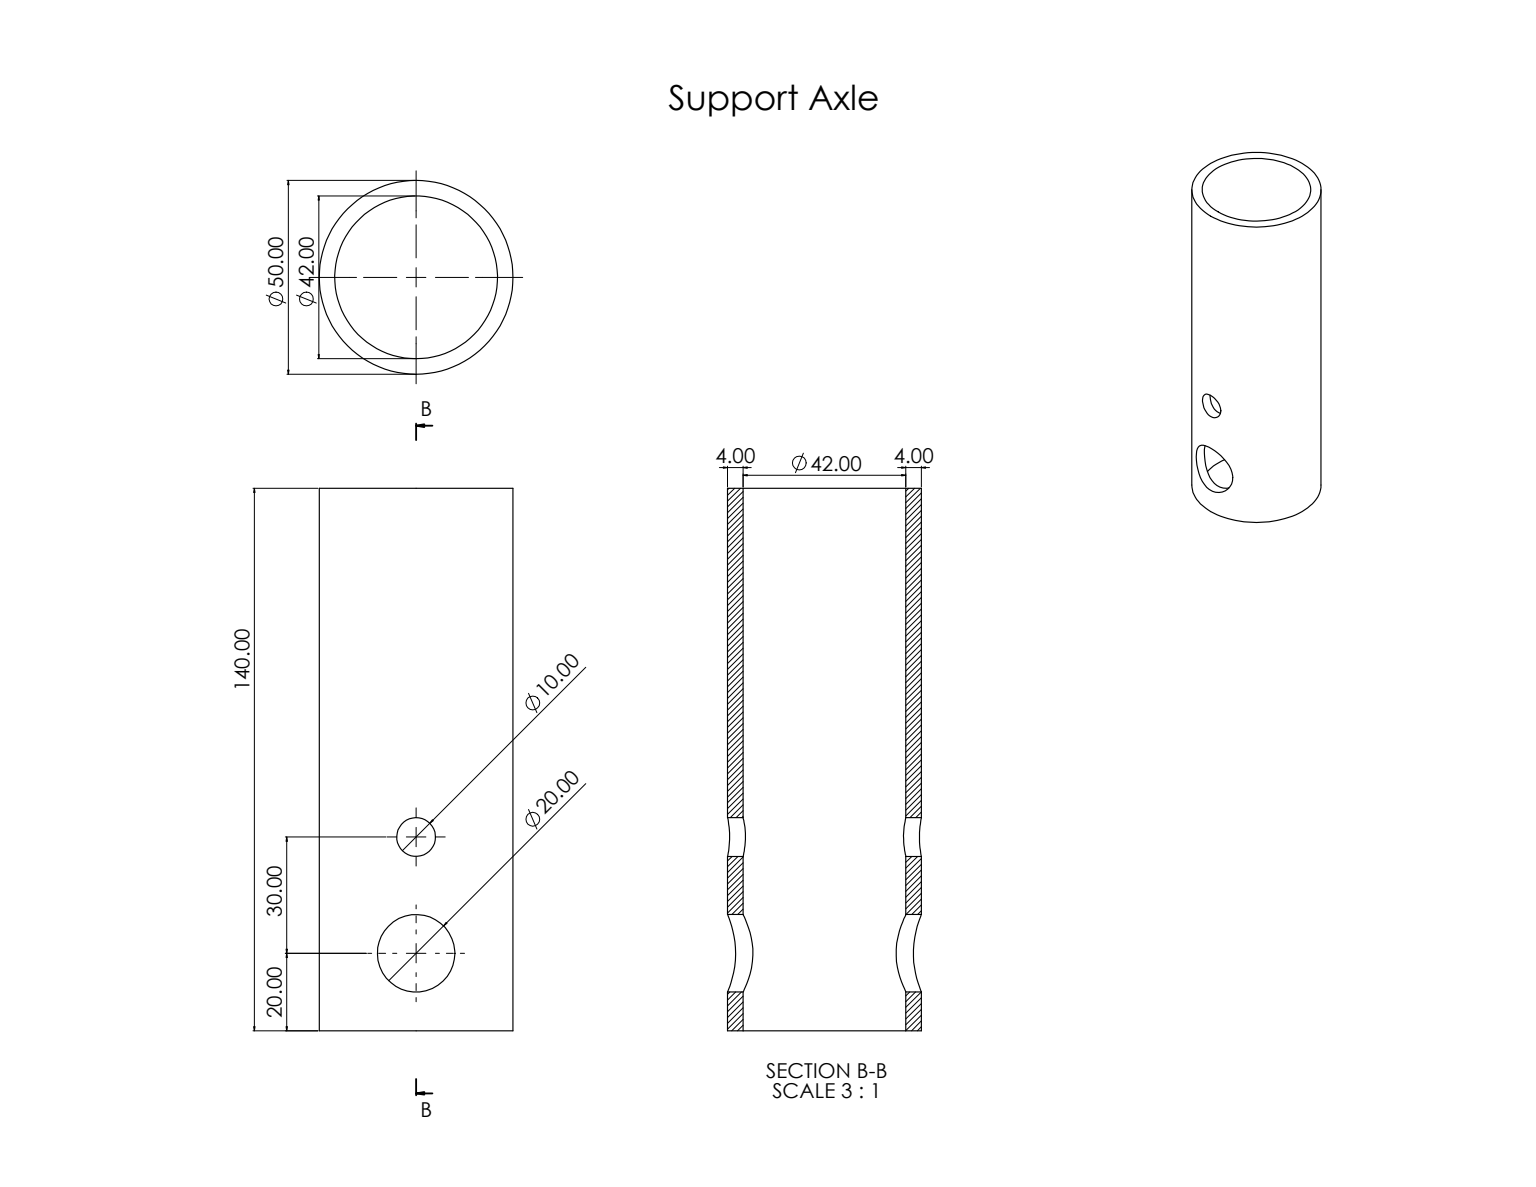
ISO-10303-21;
HEADER;
FILE_DESCRIPTION (('STEP AP214'),
    '1' );
FILE_NAME ('Support Axle.step',
    '2026-10-19T17:36:30',
    ( '' ),
    ( '' ),
    'SwSTEP 2.0',
    'SolidWorks 2025',
    '' );
FILE_SCHEMA (( 'AUTOMOTIVE_DESIGN' ));
ENDSEC;

DATA;
#26=CARTESIAN_POINT ( 'NONE',  ( 5.000000000000000888, 49.66980702654861801, -24.49489742783178059 ) ) ;
#42=CARTESIAN_POINT ( 'NONE',  ( -5.000000000000000000, 50.00000000000000000, 24.49489742783178414 ) ) ;
#55=CARTESIAN_POINT ( 'NONE',  ( 1.302272420532246455, 45.16122859629937381, -20.96210264449279137 ) ) ;
#72=DIRECTION ( 'NONE',  ( 0.000000000000000000, 0.000000000000000000, 1.000000000000000000 ) ) ;
#75=EDGE_CURVE ( 'NONE', #1856, #7546, #10580, .T. ) ;
#100=EDGE_CURVE ( 'NONE', #1932, #332, #3178, .T. ) ;
#104=CARTESIAN_POINT ( 'NONE',  ( -9.477880355945590196, 23.25612560302911902, 18.74165831626246970 ) ) ;
#120=CARTESIAN_POINT ( 'NONE',  ( -3.766911610146119305, 46.69571375074811925, -24.71569286637712892 ) ) ;
#139=EDGE_CURVE ( 'NONE', #6118, #11306, #5452, .T. ) ;
#141=EDGE_LOOP ( 'NONE', ( #2879, #8210, #6869, #7953, #8806, #9023 ) ) ;
#143=CARTESIAN_POINT ( 'NONE',  ( -3.767068525368503895, 53.30379312071067233, -24.71564595051174607 ) ) ;
#153=FACE_BOUND ( 'NONE', #206, .T. ) ;
#183=CARTESIAN_POINT ( 'NONE',  ( 4.999999999999999112, 49.83503777815744940, -20.39607805437113441 ) ) ;
#192=AXIS2_PLACEMENT_3D ( 'NONE', #3678, #11483, #9714 ) ;
#196=CIRCLE ( 'NONE', #3434, 25.00000000000000000 ) ;
#204=ORIENTED_EDGE ( 'NONE', *, *, #7341, .T. ) ;
#206=EDGE_LOOP ( 'NONE', ( #5971, #3892 ) ) ;
#207=DIRECTION ( 'NONE',  ( 1.000000000000000000, 0.000000000000000000, 0.000000000000000000 ) ) ;
#216=MECHANICAL_DESIGN_GEOMETRIC_PRESENTATION_REPRESENTATION('',(#1626),#7294);
#226=PRODUCT_DEFINITION_SHAPE ( 'NONE', 'NONE',  #5124 ) ;
#231=CARTESIAN_POINT ( 'NONE',  ( -10.00000000000000178, 20.33047844303349905, 18.46618531261938756 ) ) ;
#233=ORIENTED_EDGE ( 'NONE', *, *, #8654, .T. ) ;
#239=ORIENTED_EDGE ( 'NONE', *, *, #75, .F. ) ;
#252=CARTESIAN_POINT ( 'NONE',  ( 3.053062343563090142, 46.02672757820099037, 20.77871069257179215 ) ) ;
#281=CARTESIAN_POINT ( 'NONE',  ( 3.052678183968668524, 46.02654057254596154, -24.81443426854575307 ) ) ;
#289=PRODUCT_DEFINITION_CONTEXT ( 'detailed design', #1328, 'design' ) ;
#310=CARTESIAN_POINT ( 'NONE',  ( 8.648152576036682859, 25.03146049264868367, 19.13735728885347243 ) ) ;
#314=CARTESIAN_POINT ( 'NONE',  ( 3.974373595566621731, 46.94861671663893077, 20.62131536938402832 ) ) ;
#325=AXIS2_PLACEMENT_3D ( 'NONE', #1284, #11686, #5158 ) ;
#332=VERTEX_POINT ( 'NONE', #3766 ) ;
#349=ORIENTED_EDGE ( 'NONE', *, *, #10874, .F. ) ;
#355=CIRCLE ( 'NONE', #6829, 21.00000000000000000 ) ;
#360=ORIENTED_EDGE ( 'NONE', *, *, #5907, .F. ) ;
#369=CARTESIAN_POINT ( 'NONE',  ( 10.00000000000000533, 19.67046583110989744, -22.91287847477920181 ) ) ;
#373=DIRECTION ( 'NONE',  ( 0.000000000000000000, 0.000000000000000000, -1.000000000000000000 ) ) ;
#376=CARTESIAN_POINT ( 'NONE',  ( 3.260856397143627294, 29.47603743248158636, -20.75437471433135883 ) ) ;
#377=CARTESIAN_POINT ( 'NONE',  ( 1.612540704446980389, 45.26432593853714081, 20.93858753690425090 ) ) ;
#384=AXIS2_PLACEMENT_3D ( 'NONE', #11930, #5963, #3236 ) ;
#398=CARTESIAN_POINT ( 'NONE',  ( 2.571758278209441661E-15, 0.000000000000000000, 21.00000000000000000 ) ) ;
#426=ORIENTED_EDGE ( 'NONE', *, *, #9632, .F. ) ;
#427=CARTESIAN_POINT ( 'NONE',  ( -6.613021203892899713, 12.47133511838782383, -19.93742635182809053 ) ) ;
#428=CARTESIAN_POINT ( 'NONE',  ( -0.3295322344531997905, 30.00000000000001066, 25.00000000000001066 ) ) ;
#442=CARTESIAN_POINT ( 'NONE',  ( 3.974960981574284347, 46.94936902441865101, 24.68265737646872893 ) ) ;
#447=CARTESIAN_POINT ( 'NONE',  ( 0.000000000000000000, 139.9999999999999716, 0.000000000000000000 ) ) ;
#467=ORIENTED_EDGE ( 'NONE', *, *, #7068, .F. ) ;
#468=CYLINDRICAL_SURFACE ( 'NONE', #9354, 5.000000000000000000 ) ;
#489=CARTESIAN_POINT ( 'NONE',  ( 9.917674697986294419, 18.67684296126092747, -22.94866065126248600 ) ) ;
#494=CARTESIAN_POINT ( 'NONE',  ( 3.061616998149962604E-15, 10.00000000000000000, 25.00000000000000000 ) ) ;
#500=CARTESIAN_POINT ( 'NONE',  ( 2.612127725832936065, 29.65839247515747346, 24.86517017815632968 ) ) ;
#517=VECTOR ( 'NONE', #12407, 1000.000000000000000 ) ;
#529=CARTESIAN_POINT ( 'NONE',  ( -2.067585255946370548, 45.44456205236168245, 24.91481882275639848 ) ) ;
#544=ORIENTED_EDGE ( 'NONE', *, *, #6668, .F. ) ;
#548=CARTESIAN_POINT ( 'NONE',  ( -2.620496854523448604, 10.32661740714168097, -24.87086379260451707 ) ) ;
#550=CARTESIAN_POINT ( 'NONE',  ( 6.615773601782837687, 12.47291401044366310, -24.11353245396511014 ) ) ;
#555=DIRECTION ( 'NONE',  ( 1.000000000000000000, 0.000000000000000000, 0.000000000000000000 ) ) ;
#558=CARTESIAN_POINT ( 'NONE',  ( -1.614380680224908104, 54.74360302825979119, 24.94967786989446878 ) ) ;
#573=LINE ( 'NONE', #5584, #10338 ) ;
#597=LINE ( 'NONE', #3505, #11293 ) ;
#610=CARTESIAN_POINT ( 'NONE',  ( -7.514688383768903357, 13.39426057884744026, -23.84485093628785535 ) ) ;
#611=CARTESIAN_POINT ( 'NONE',  ( 2.620611987601386250, 10.32688167823381953, -24.87076294850758984 ) ) ;
#616=CARTESIAN_POINT ( 'NONE',  ( 5.000000000000000888, 50.00000000000000000, -20.39607805437114152 ) ) ;
#621=CARTESIAN_POINT ( 'NONE',  ( 4.444397983376138228, 28.96407317687630822, 24.60352964329958070 ) ) ;
#622=CARTESIAN_POINT ( 'NONE',  ( -4.839306774598123084, 51.30008082132634684, 24.52723862394605092 ) ) ;
#640=EDGE_CURVE ( 'NONE', #4818, #9118, #196, .T. ) ;
#646=CARTESIAN_POINT ( 'NONE',  ( -1.322110193236855746, 29.91777919888772885, 20.96095187701988394 ) ) ;
#653=CARTESIAN_POINT ( 'NONE',  ( 3.561025220032636440, 10.64985055133391079, 20.69813086000296209 ) ) ;
#666=( NAMED_UNIT ( * ) SI_UNIT ( $, .STERADIAN. ) SOLID_ANGLE_UNIT ( ) );
#670=CARTESIAN_POINT ( 'NONE',  ( -3.245616027290198602, 10.51897860477085622, -24.79588311023535852 ) ) ;
#671=CARTESIAN_POINT ( 'NONE',  ( 9.917815328463536417, 18.67816480429018711, -18.51049262088216807 ) ) ;
#677=CARTESIAN_POINT ( 'NONE',  ( 0.000000000000000000, 139.9999999999999716, 0.000000000000000000 ) ) ;
#705=CARTESIAN_POINT ( 'NONE',  ( -5.310537848405668448, 28.47956428665436235, 20.31934704339811049 ) ) ;
#723=CARTESIAN_POINT ( 'NONE',  ( -3.554546826686217020, 29.35267307038308360, -24.74790415999775917 ) ) ;
#731=CARTESIAN_POINT ( 'NONE',  ( 2.218782135151963431, 54.49261812855775844, 20.88465242318871873 ) ) ;
#741=CARTESIAN_POINT ( 'NONE',  ( 9.657343816332662811, 22.61594140643868300, 23.05962942824199757 ) ) ;
#746=CARTESIAN_POINT ( 'NONE',  ( -3.255620798467798060, 29.46102596484070446, -20.74857864660710405 ) ) ;
#747=EDGE_CURVE ( 'NONE', #3111, #7940, #4337, .T. ) ;
#769=CARTESIAN_POINT ( 'NONE',  ( -5.000000000000000000, 50.00000000000000000, -20.39607805437114152 ) ) ;
#772=CARTESIAN_POINT ( 'NONE',  ( 9.932934464065827029, 18.66923383145512005, 18.50293221336126237 ) ) ;
#775=CARTESIAN_POINT ( 'NONE',  ( -0.6569842770428546697, 54.96739046863824996, -24.99342020365237360 ) ) ;
#794=CARTESIAN_POINT ( 'NONE',  ( 6.113716319958878209, 12.07992478634019662, -20.09207169644096780 ) ) ;
#797=ADVANCED_FACE ( 'NONE', ( #11879 ), #3185, .F. ) ;
#808=CARTESIAN_POINT ( 'NONE',  ( 1.342157722727130131E-15, 30.00000000000002132, -21.00000000000000355 ) ) ;
#829=ORIENTED_EDGE ( 'NONE', *, *, #2173, .T. ) ;
#855=CARTESIAN_POINT ( 'NONE',  ( 0.6627065662273624591, 10.01637405127483049, -20.99218728179891613 ) ) ;
#859=CARTESIAN_POINT ( 'NONE',  ( -3.305497356469124792, 46.23421970496524125, 20.73954946919153031 ) ) ;
#866=CARTESIAN_POINT ( 'NONE',  ( 5.000000000000000888, 50.00000000000000000, -20.39607805437114152 ) ) ;
#872=CARTESIAN_POINT ( 'NONE',  ( 0.000000000000000000, 0.000000000000000000, 0.000000000000000000 ) ) ;
#877=CARTESIAN_POINT ( 'NONE',  ( -3.051621101708449579, 53.97419359098365987, -20.77889715443343377 ) ) ;
#878=CARTESIAN_POINT ( 'NONE',  ( 3.061616997868383043E-15, 139.9999999999999716, 25.00000000000000000 ) ) ;
#892=B_SPLINE_CURVE_WITH_KNOTS ( 'NONE', 3,
 ( #7213, #5385, #9191, #2454, #500, #2580, #12107, #6328, #621, #5570, #3473, #6450, #6268, #8421, #9439, #12291, #6510, #11087, #1687, #10141, #10312, #741, #4609, #5321, #1631, #4364, #9318, #8299 ),
 .UNSPECIFIED., .F., .F.,
 ( 4, 2, 2, 2, 2, 2, 2, 2, 2, 2, 2, 2, 2, 4 ),
 ( 0.04738593773884331589, 0.04935840384251231894, 0.05034463689434681699, 0.05133086994618132198, 0.05231710299801582004, 0.05330333604985031809, 0.05527580215351931420, 0.05626203520535381225, 0.05724826825718831030, 0.05922073436085731335, 0.06020696741269181834, 0.06119320046452632333, 0.06217943351636082833, 0.06316566656819533332 ),
 .UNSPECIFIED. ) ;
#917=CARTESIAN_POINT ( 'NONE',  ( 8.667518415056527203, 14.97026592263945410, 23.45254893740142066 ) ) ;
#924=CARTESIAN_POINT ( 'NONE',  ( 0.3308316500937774629, 9.999999999999994671, -21.00000000000000711 ) ) ;
#937=ORIENTED_EDGE ( 'NONE', *, *, #4287, .F. ) ;
#941=CARTESIAN_POINT ( 'NONE',  ( -4.473766101552917540, 28.96742557902637927, -20.52713491992151162 ) ) ;
#946=DIRECTION ( 'NONE',  ( -0.000000000000000000, -1.000000000000000000, -0.000000000000000000 ) ) ;
#950=CARTESIAN_POINT ( 'NONE',  ( 1.326742001580319741, 29.91711497655587948, -24.96694321103489855 ) ) ;
#951=UNCERTAINTY_MEASURE_WITH_UNIT (LENGTH_MEASURE( 1.000000000000000082E-05 ), #4583, 'distance_accuracy_value', 'NONE');
#958=EDGE_CURVE ( 'NONE', #8162, #11970, #11300, .T. ) ;
#963=ORIENTED_EDGE ( 'NONE', *, *, #640, .T. ) ;
#978=CARTESIAN_POINT ( 'NONE',  ( -6.849710128414980836, 27.29284600759404356, -24.04449974210336904 ) ) ;
#980=ORIENTED_EDGE ( 'NONE', *, *, #75, .T. ) ;
#982=CARTESIAN_POINT ( 'NONE',  ( 6.110979747148361341, 12.05740682582580625, 24.24803741642852373 ) ) ;
#985=EDGE_CURVE ( 'NONE', #8822, #6118, #9067, .T. ) ;
#987=FACE_OUTER_BOUND ( 'NONE', #9258, .T. ) ;
#1002=CARTESIAN_POINT ( 'NONE',  ( 3.975237584097107923, 53.05037957731131826, -20.62115343197593020 ) ) ;
#1016=CARTESIAN_POINT ( 'NONE',  ( 10.00000000000000178, 20.33006360438132987, -18.46618531261938756 ) ) ;
#1020=CARTESIAN_POINT ( 'NONE',  ( 6.844556472468130259, 27.29775667647069071, -24.04598060202682319 ) ) ;
#1044=DIRECTION ( 'NONE',  ( -0.000000000000000000, -1.000000000000000000, -0.000000000000000000 ) ) ;
#1059=CARTESIAN_POINT ( 'NONE',  ( -9.983660626454435416, 20.66196728388187864, 18.47506278258854806 ) ) ;
#1071=CARTESIAN_POINT ( 'NONE',  ( -5.000000000000000000, 50.00000000000000000, -24.49489742783178059 ) ) ;
#1072=CARTESIAN_POINT ( 'NONE',  ( 4.490871182873028111, 47.77729020916527958, -20.51460075614775036 ) ) ;
#1106=AXIS2_PLACEMENT_3D ( 'NONE', #12286, #5873, #10807 ) ;
#1109=CARTESIAN_POINT ( 'NONE',  ( 4.491542451266983704, 47.77873343313099497, -24.59354576118897739 ) ) ;
#1114=DIRECTION ( 'NONE',  ( 1.000000000000000000, 0.000000000000000000, 0.000000000000000000 ) ) ;
#1125=CARTESIAN_POINT ( 'NONE',  ( 4.999999999999999112, 50.32998418051842293, -24.49489742783177348 ) ) ;
#1130=ORIENTED_EDGE ( 'NONE', *, *, #3730, .T. ) ;
#1133=CYLINDRICAL_SURFACE ( 'NONE', #4793, 25.00000000000000000 ) ;
#1138=CARTESIAN_POINT ( 'NONE',  ( 9.477187959615639201, 23.25714206674319939, 18.74197276232252563 ) ) ;
#1144=CARTESIAN_POINT ( 'NONE',  ( 9.658351069856484727, 22.61227114741398836, -23.05920763558311037 ) ) ;
#1147=PRODUCT_CONTEXT ( 'NONE', #8453, 'mechanical' ) ;
#1174=EDGE_CURVE ( 'NONE', #8715, #3634, #892, .T. ) ;
#1176=CARTESIAN_POINT ( 'NONE',  ( 2.065847364689658683, 45.44381439048179772, -24.91495664786098274 ) ) ;
#1178=ORIENTED_EDGE ( 'NONE', *, *, #6560, .F. ) ;
#1199=DIRECTION ( 'NONE',  ( 0.000000000000000000, 0.000000000000000000, 1.000000000000000000 ) ) ;
#1202=CARTESIAN_POINT ( 'NONE',  ( 8.957304208062865314, 24.45789625178892734, 18.99462261546309705 ) ) ;
#1221=VERTEX_POINT ( 'NONE', #7338 ) ;
#1254=CARTESIAN_POINT ( 'NONE',  ( -4.158535434072708092, 10.89987024370912572, -20.58639742492232827 ) ) ;
#1259=CARTESIAN_POINT ( 'NONE',  ( 2.630514865864268970, 29.67066479083239372, 20.84486189436999837 ) ) ;
#1260=CARTESIAN_POINT ( 'NONE',  ( 3.975399702753076525, 46.95009918027220408, -20.62111044216656452 ) ) ;
#1265=ORIENTED_EDGE ( 'NONE', *, *, #2271, .T. ) ;
#1266=B_SPLINE_CURVE_WITH_KNOTS ( 'NONE', 3,
 ( #4749, #8741, #6707, #55, #8495, #2843, #5641, #3668, #10576, #1887, #1260, #9763, #1072, #5952, #10828, #9827, #6896, #11726, #183, #10761 ),
 .UNSPECIFIED., .F., .F.,
 ( 4, 2, 2, 2, 2, 2, 2, 2, 2, 4 ),
 ( 0.01568878760782931384, 0.01666929802245319808, 0.01764980843707708580, 0.01863031885170097005, 0.01961082926632485429, 0.02059133968094873854, 0.02157185009557262279, 0.02255236051019651050, 0.02304261571750846130, 0.02353287092482041556 ),
 .UNSPECIFIED. ) ;
#1280=ORIENTED_EDGE ( 'NONE', *, *, #3433, .T. ) ;
#1284=CARTESIAN_POINT ( 'NONE',  ( 0.000000000000000000, 20.00000000000000355, -28.00000000000000711 ) ) ;
#1297=CARTESIAN_POINT ( 'NONE',  ( 1.302738838705299829, 54.83847614797452508, -20.96203534374045674 ) ) ;
#1299=ORIENTED_EDGE ( 'NONE', *, *, #9071, .F. ) ;
#1319=CARTESIAN_POINT ( 'NONE',  ( -6.116903510341333394, 12.06222645458920084, -20.09722343790940613 ) ) ;
#1322=CARTESIAN_POINT ( 'NONE',  ( -8.658175568303594360, 14.98574592473889311, 23.45342671841680371 ) ) ;
#1324=CARTESIAN_POINT ( 'NONE',  ( -3.050580840359966128, 46.02510565206127779, -24.81467268664276560 ) ) ;
#1328=APPLICATION_CONTEXT ( 'automotive_design' ) ;
#1380=CARTESIAN_POINT ( 'NONE',  ( -7.294862588765995248, 13.15250477205630553, -19.69373592174549259 ) ) ;
#1412=ADVANCED_FACE ( 'NONE', ( #11714 ), #7907, .F. ) ;
#1441=DIRECTION ( 'NONE',  ( -0.000000000000000000, -1.000000000000000000, -0.000000000000000000 ) ) ;
#1444=CARTESIAN_POINT ( 'NONE',  ( -3.558434346354896416, 10.64888650799004033, -20.69856808805790038 ) ) ;
#1450=CARTESIAN_POINT ( 'NONE',  ( -9.463516830393745138, 16.75202061662974273, 18.74709386869566430 ) ) ;
#1455=VECTOR ( 'NONE', #6408, 1000.000000000000000 ) ;
#1480=DIRECTION ( 'NONE',  ( 0.000000000000000000, 0.000000000000000000, 1.000000000000000000 ) ) ;
#1482=VECTOR ( 'NONE', #5857, 1000.000000000000000 ) ;
#1498=CARTESIAN_POINT ( 'NONE',  ( -4.441326820874226478, 11.03441940688963108, -24.60408056175351987 ) ) ;
#1500=CARTESIAN_POINT ( 'NONE',  ( -9.103371648737914157, 24.15160165414906857, 23.28405058525132176 ) ) ;
#1506=CARTESIAN_POINT ( 'NONE',  ( -8.488010075893786421, 14.70289628708776242, 19.20917730135813528 ) ) ;
#1514=CARTESIAN_POINT ( 'NONE',  ( 3.298734236876446957, 53.76100060739371145, 24.78173945428942204 ) ) ;
#1536=AXIS2_PLACEMENT_3D ( 'NONE', #5941, #8037, #8854 ) ;
#1565=CARTESIAN_POINT ( 'NONE',  ( 8.486510062750307171, 14.70060591898896618, -23.51628241912814588 ) ) ;
#1593=AXIS2_PLACEMENT_3D ( 'NONE', #10131, #1441, #4352 ) ;
#1600=CARTESIAN_POINT ( 'NONE',  ( -1.614021781250221999, 45.25640150583762988, -20.94007668992154692 ) ) ;
#1604=( NAMED_UNIT ( * ) PLANE_ANGLE_UNIT ( ) SI_UNIT ( $, .RADIAN. ) );
#1621=CARTESIAN_POINT ( 'NONE',  ( 9.105349949761121664, 15.85277269881838258, -23.28327519851026040 ) ) ;
#1626=STYLED_ITEM('',(#12584),#2150);
#1628=CARTESIAN_POINT ( 'NONE',  ( -7.537341967019228761, 13.39683431484485965, 19.60665308794510864 ) ) ;
#1631=CARTESIAN_POINT ( 'NONE',  ( 9.916835782772588814, 21.32911185711201796, 22.94902338049798374 ) ) ;
#1676=ORIENTED_EDGE ( 'NONE', *, *, #10874, .T. ) ;
#1678=CARTESIAN_POINT ( 'NONE',  ( -8.664197377259947430, 14.96499702975700608, -23.45374477514955203 ) ) ;
#1679=CARTESIAN_POINT ( 'NONE',  ( 10.00000000000000711, 19.66959671226640793, -18.46618531261938756 ) ) ;
#1683=CARTESIAN_POINT ( 'NONE',  ( -0.3273843838414227103, 45.00000000000000711, 20.99999999999999645 ) ) ;
#1687=CARTESIAN_POINT ( 'NONE',  ( 8.972329510183547185, 24.46440230363330315, 23.33606587946024291 ) ) ;
#1722=CARTESIAN_POINT ( 'NONE',  ( -6.197539731915355238E-14, 9.999999999999182876, 21.00000000000039080 ) ) ;
#1740=CARTESIAN_POINT ( 'NONE',  ( 1.659095203930551543, 10.13304969779982301, -20.93688979605049738 ) ) ;
#1776=CARTESIAN_POINT ( 'NONE',  ( -5.000000000000000888, 49.67263425446288494, -20.39607805437114152 ) ) ;
#1778=B_SPLINE_CURVE_WITH_KNOTS ( 'NONE', 3,
 ( #9551, #9365, #8407, #9609, #6556, #8526, #9488, #5615, #917, #3576, #8650, #11322, #2629, #7578, #982, #4848, #9798, #6929, #4912, #1918, #8967, #8714, #6871, #3003 ),
 .UNSPECIFIED., .F., .F.,
 ( 4, 2, 2, 2, 2, 2, 2, 2, 2, 2, 2, 4 ),
 ( 0.000000000000000000, 0.001975470015275241145, 0.002963205022912861284, 0.003950940030550481423, 0.005926410045825732976, 0.006914145053463355284, 0.007901880061100976724, 0.009877350076376223073, 0.01185282009165146769, 0.01284055509928909086, 0.01382829010692671404, 0.01580376012220196039 ),
 .UNSPECIFIED. ) ;
#1779=CARTESIAN_POINT ( 'NONE',  ( 9.737577724063894991, 17.70041058371123555, 18.60604745661291659 ) ) ;
#1784=ADVANCED_FACE ( 'NONE', ( #6253 ), #5244, .T. ) ;
#1788=CARTESIAN_POINT ( 'NONE',  ( 5.000000000000000000, 50.00000000000000000, -24.49489742783178414 ) ) ;
#1827=FACE_OUTER_BOUND ( 'NONE', #6135, .T. ) ;
#1839=EDGE_LOOP ( 'NONE', ( #11508, #2743, #7233, #12183, #8498, #2835, #829, #9052, #10546, #10410, #9366, #12012, #9085, #9441, #6536, #8348 ) ) ;
#1843=CARTESIAN_POINT ( 'NONE',  ( 7.513991638149614793, 13.39363280574569792, 19.61093064431749156 ) ) ;
#1856=VERTEX_POINT ( 'NONE', #5970 ) ;
#1864=CARTESIAN_POINT ( 'NONE',  ( 3.061617454482527662E-15, 30.00000000000001066, 25.00000000000000000 ) ) ;
#1887=CARTESIAN_POINT ( 'NONE',  ( 3.765166081389465624, 46.69397311189987931, -20.66103212045354098 ) ) ;
#1918=CARTESIAN_POINT ( 'NONE',  ( 2.610381677634093123, 10.34108370468245219, 24.86537221636008965 ) ) ;
#1932=VERTEX_POINT ( 'NONE', #5056 ) ;
#1940=CARTESIAN_POINT ( 'NONE',  ( 4.492685090163540451, 52.21864068105092116, -20.51419621738226695 ) ) ;
#1948=CARTESIAN_POINT ( 'NONE',  ( -0.3317315395883421170, 55.00000000000000711, -21.00000000000000000 ) ) ;
#1967=AXIS2_PLACEMENT_3D ( 'NONE', #3895, #3202, #1114 ) ;
#1988=CARTESIAN_POINT ( 'NONE',  ( 0.000000000000000000, 139.9999999999999716, -25.00000000000000000 ) ) ;
#1993=CARTESIAN_POINT ( 'NONE',  ( -10.00000000000000355, 20.00000000000000355, 18.46618531261938756 ) ) ;
#2007=CARTESIAN_POINT ( 'NONE',  ( 0.000000000000000000, 0.000000000000000000, 0.000000000000000000 ) ) ;
#2011=CARTESIAN_POINT ( 'NONE',  ( 1.653699482248477182, 29.86790856825577478, 20.93734097219926582 ) ) ;
#2028=CIRCLE ( 'NONE', #12370, 25.00000000000000000 ) ;
#2044=VERTEX_POINT ( 'NONE', #5183 ) ;
#2061=ORIENTED_EDGE ( 'NONE', *, *, #4367, .F. ) ;
#2073=CARTESIAN_POINT ( 'NONE',  ( 2.636325768737970421, 29.66875067697592883, -20.84397515108148724 ) ) ;
#2078=CARTESIAN_POINT ( 'NONE',  ( 10.00000000000000355, 20.00000000000000355, -22.91287847477919826 ) ) ;
#2106=CARTESIAN_POINT ( 'NONE',  ( -10.00000000000000533, 20.66054119461773553, -22.91287847477919470 ) ) ;
#2109=AXIS2_PLACEMENT_3D ( 'NONE', #447, #4560, #11286 ) ;
#2124=EDGE_LOOP ( 'NONE', ( #4978, #8968, #10794, #2582, #3424, #204, #9766, #4611, #9474, #963, #4270, #1676, #233, #7725, #1265, #2770 ) ) ;
#2126=CARTESIAN_POINT ( 'NONE',  ( 2.221110608488543026, 54.49139573732541209, -24.90296241992962578 ) ) ;
#2140=CARTESIAN_POINT ( 'NONE',  ( 9.931121997304011018, 21.34393702597181530, 18.50391133509319630 ) ) ;
#2141=CARTESIAN_POINT ( 'NONE',  ( -1.614845647245295668, 54.74348708565381827, 20.94004496404980742 ) ) ;
#2145=CARTESIAN_POINT ( 'NONE',  ( 4.999999999999999112, 49.66826422043975242, 20.39607805437114507 ) ) ;
#2147=CARTESIAN_POINT ( 'NONE',  ( 9.104442389086463194, 24.14915179589751304, -23.28362858151144721 ) ) ;
#2150=MANIFOLD_SOLID_BREP ( 'Cut-Extrude1[1]', #9310 ) ;
#2166=CARTESIAN_POINT ( 'NONE',  ( -3.973726775714538029, 53.05247132632594287, -24.68286527305685141 ) ) ;
#2173=EDGE_CURVE ( 'NONE', #3634, #9164, #1778, .T. ) ;
#2180=EDGE_LOOP ( 'NONE', ( #6946, #7322, #9894, #5335, #11443, #10716 ) ) ;
#2181=CARTESIAN_POINT ( 'NONE',  ( 0.6582936873354101603, 54.96735637312282563, -20.99215814668205482 ) ) ;
#2186=LINE ( 'NONE', #1988, #5156 ) ;
#2201=EDGE_CURVE ( 'NONE', #2752, #10467, #5726, .T. ) ;
#2204=CARTESIAN_POINT ( 'NONE',  ( -9.461967865576259129, 16.74741879838144598, -18.74787822604630350 ) ) ;
#2211=CARTESIAN_POINT ( 'NONE',  ( 10.00000000000000355, 20.00000000000000355, 18.46618531261938401 ) ) ;
#2212=CARTESIAN_POINT ( 'NONE',  ( -2.222896043811084077, 54.49078271291326558, 20.88425106962813516 ) ) ;
#2217=CARTESIAN_POINT ( 'NONE',  ( 3.304159235005521111, 46.23328646880356274, 20.73974243245384841 ) ) ;
#2233=ORIENTED_EDGE ( 'NONE', *, *, #8936, .T. ) ;
#2234=ORIENTED_EDGE ( 'NONE', *, *, #3811, .T. ) ;
#2248=CARTESIAN_POINT ( 'NONE',  ( -3.304393266822325703, 46.23318141187127139, 24.78176792680001839 ) ) ;
#2268=CARTESIAN_POINT ( 'NONE',  ( -3.251483927478052482, 10.53766038749295753, -20.74918120701668300 ) ) ;
#2271=EDGE_CURVE ( 'NONE', #5152, #7013, #6332, .T. ) ;
#2274=CARTESIAN_POINT ( 'NONE',  ( -2.509809017951089682, 45.66333224303983229, -24.87518608377025231 ) ) ;
#2275=CARTESIAN_POINT ( 'NONE',  ( -0.3310653830415872800, 54.99172937625127133, 20.99802641299722339 ) ) ;
#2306=CARTESIAN_POINT ( 'NONE',  ( -5.000000000000000000, 50.00000000000000000, 24.49489742783178414 ) ) ;
#2318=B_SPLINE_CURVE_WITH_KNOTS ( 'NONE', 3,
 ( #11987, #4369, #3415, #7284, #2459, #6335, #10202, #9324, #8364, #1514, #8306, #12174, #3477, #7409, #6151, #2525, #5455, #10026, #8118, #6515 ),
 .UNSPECIFIED., .F., .F.,
 ( 4, 2, 2, 2, 2, 2, 2, 2, 2, 4 ),
 ( 0.02350813035260379893, 0.02448705762280033518, 0.02546598489299686796, 0.02644491216319340421, 0.02693437579829167233, 0.02742383943338994046, 0.02840276670358647670, 0.02938169397378300948, 0.03036062124397954226, 0.03133954851417607851 ),
 .UNSPECIFIED. ) ;
#2329=CARTESIAN_POINT ( 'NONE',  ( -7.519134213638725583, 26.60056234660722652, 23.84343405217310874 ) ) ;
#2333=DIRECTION ( 'NONE',  ( -0.000000000000000000, -0.000000000000000000, 1.000000000000000000 ) ) ;
#2335=CARTESIAN_POINT ( 'NONE',  ( -10.00000000000000355, 19.33860219128660063, 18.46618531261938045 ) ) ;
#2338=CARTESIAN_POINT ( 'NONE',  ( 2.506524500420500345, 45.66117316082983990, 20.85169879525578907 ) ) ;
#2364=VERTEX_POINT ( 'NONE', #3618 ) ;
#2385=CARTESIAN_POINT ( 'NONE',  ( -4.451684831872904091, 11.03962932791216112, -20.52483624935579343 ) ) ;
#2386=CARTESIAN_POINT ( 'NONE',  ( -5.303430480311382311, 28.48399989248413178, 24.43255084236253794 ) ) ;
#2388=CARTESIAN_POINT ( 'NONE',  ( -10.00000000000000355, 20.00000000000000355, 22.91287847477919826 ) ) ;
#2397=CARTESIAN_POINT ( 'NONE',  ( 0.3271393060908659445, 45.00000000000000711, 25.00000000000000355 ) ) ;
#2398=EDGE_CURVE ( 'NONE', #11698, #2695, #4652, .T. ) ;
#2424=CARTESIAN_POINT ( 'NONE',  ( -1.612909136089518691, 45.25592802960594696, 24.94976847917136453 ) ) ;
#2444=VERTEX_POINT ( 'NONE', #12444 ) ;
#2449=CARTESIAN_POINT ( 'NONE',  ( -9.869611566543289527, 18.35654797443324782, 22.96945393929722457 ) ) ;
#2454=CARTESIAN_POINT ( 'NONE',  ( 2.290457103807213457, 29.73981914200485477, 24.89699738223682246 ) ) ;
#2455=CARTESIAN_POINT ( 'NONE',  ( 0.000000000000000000, 139.9999999999999716, 0.000000000000000000 ) ) ;
#2458=CARTESIAN_POINT ( 'NONE',  ( 4.491750101222253377, 47.77928715861156661, 24.59350609687774281 ) ) ;
#2459=CARTESIAN_POINT ( 'NONE',  ( 1.614235646224727372, 54.74352724365349587, 24.94966740611544509 ) ) ;
#2466=B_SPLINE_CURVE_WITH_KNOTS ( 'NONE', 3,
 ( #11905, #1125, #8917, #7969, #3968, #6004, #8789, #8035, #6944, #7843, #5877, #3017, #10811, #6883, #2126, #7073, #6069, #9876, #5814, #4862 ),
 .UNSPECIFIED., .F., .F.,
 ( 4, 2, 2, 2, 2, 2, 2, 2, 2, 4 ),
 ( 0.02350824016915415912, 0.02448716854195917558, 0.02546609691476419204, 0.02644502528756920851, 0.02693448947397171500, 0.02742395366037422497, 0.02840288203317925531, 0.02938181040598428218, 0.03036073877878931251, 0.03133966715159434285 ),
 .UNSPECIFIED. ) ;
#2484=CARTESIAN_POINT ( 'NONE',  ( -3.051014581595654640, 46.02544827001062089, 24.81461801464184802 ) ) ;
#2493=B_SPLINE_CURVE_WITH_KNOTS ( 'NONE', 3,
 ( #8522, #3757, #6611, #4591, #9422, #9483, #723, #7637, #8463, #11502, #10544, #6046, #978, #7698, #6925, #10863, #4008, #8710, #8898, #7885, #10792, #5922, #2106, #12518 ),
 .UNSPECIFIED., .F., .F.,
 ( 4, 2, 2, 2, 2, 2, 2, 2, 2, 2, 2, 4 ),
 ( 5.438949063372056100E-19, 0.001975691086292785757, 0.002963536629439178418, 0.003951382172585572380, 0.005927073258878355969, 0.006914918802024747763, 0.007902764345171137822, 0.009878455431463928349, 0.01185414651775671888, 0.01284199206090311240, 0.01382983760404950767, 0.01580552869034228605 ),
 .UNSPECIFIED. ) ;
#2509=CARTESIAN_POINT ( 'NONE',  ( -10.00000000000000355, 20.00000000000000355, -22.91287847477919826 ) ) ;
#2511=CARTESIAN_POINT ( 'NONE',  ( -9.481431770954213079, 23.24517152888003224, 23.13387126485941536 ) ) ;
#2515=CARTESIAN_POINT ( 'NONE',  ( -1.652347697333065968, 10.13198208422932467, 24.94742907234073215 ) ) ;
#2524=VECTOR ( 'NONE', #4458, 1000.000000000000000 ) ;
#2525=CARTESIAN_POINT ( 'NONE',  ( 4.741482771685880948, 51.61996731904482516, 24.54657867284130646 ) ) ;
#2567=CARTESIAN_POINT ( 'NONE',  ( 0.6549955759030559044, 54.96769473000979644, 20.99223993983284586 ) ) ;
#2574=CARTESIAN_POINT ( 'NONE',  ( -5.000000000000000000, 49.67307781155022894, 20.39607805437114507 ) ) ;
#2575=CARTESIAN_POINT ( 'NONE',  ( -9.352703157270289225, 16.44582563935068009, 18.80282705866110149 ) ) ;
#2580=CARTESIAN_POINT ( 'NONE',  ( 3.239919941357241040, 29.46629152487073000, 24.79118428027058840 ) ) ;
#2581=CARTESIAN_POINT ( 'NONE',  ( -4.743460743378065558, 51.61424263853129446, 24.54619549801029166 ) ) ;
#2582=ORIENTED_EDGE ( 'NONE', *, *, #747, .T. ) ;
#2629=CARTESIAN_POINT ( 'NONE',  ( 7.297088297540795132, 13.15481214220262274, 23.91253034306283354 ) ) ;
#2635=CARTESIAN_POINT ( 'NONE',  ( 3.763812309688671753, 53.30741636328656341, 20.66126648110244801 ) ) ;
#2636=CARTESIAN_POINT ( 'NONE',  ( 9.670754941354928746, 17.37006389387946470, -18.64131299320824198 ) ) ;
#2640=DIRECTION ( 'NONE',  ( -0.000000000000000000, -1.000000000000000000, -0.000000000000000000 ) ) ;
#2647=ORIENTED_EDGE ( 'NONE', *, *, #10368, .T. ) ;
#2658=FACE_OUTER_BOUND ( 'NONE', #10327, .T. ) ;
#2675=CARTESIAN_POINT ( 'NONE',  ( 3.024050948510435495E-21, 45.00000000000000711, -21.00000000000000000 ) ) ;
#2677=CARTESIAN_POINT ( 'NONE',  ( 9.656537145003039058, 17.38065509551421073, 18.64841052569367719 ) ) ;
#2680=CARTESIAN_POINT ( 'NONE',  ( -0.3313438815916917579, 54.99999999999998579, -25.00000000000000000 ) ) ;
#2695=VERTEX_POINT ( 'NONE', #10589 ) ;
#2696=CARTESIAN_POINT ( 'NONE',  ( 4.967355519288257248, 50.65829285064151577, 20.40416061862378072 ) ) ;
#2697=CARTESIAN_POINT ( 'NONE',  ( 4.171089004654445986, 10.90545738055656066, -20.58391839369968324 ) ) ;
#2701=LINE ( 'NONE', #11336, #3226 ) ;
#2712=CARTESIAN_POINT ( 'NONE',  ( -10.00000000000000888, 20.66452866687815160, -18.46618531261939822 ) ) ;
#2720=CARTESIAN_POINT ( 'NONE',  ( -1.616912260125061618, 54.74267540711069557, -20.93986429502791324 ) ) ;
#2736=VERTEX_POINT ( 'NONE', #11163 ) ;
#2743=ORIENTED_EDGE ( 'NONE', *, *, #4161, .T. ) ;
#2744=DIRECTION ( 'NONE',  ( 0.000000000000000000, 0.000000000000000000, 1.000000000000000000 ) ) ;
#2752=VERTEX_POINT ( 'NONE', #8128 ) ;
#2769=CARTESIAN_POINT ( 'NONE',  ( 3.766346521502939471, 53.30452959794249068, -20.66080266315259806 ) ) ;
#2770=ORIENTED_EDGE ( 'NONE', *, *, #3384, .T. ) ;
#2773=CARTESIAN_POINT ( 'NONE',  ( -7.307805827056473191, 26.83368120074001695, -19.68893203084326515 ) ) ;
#2778=CARTESIAN_POINT ( 'NONE',  ( -1.298576428593012810, 54.83947011521958359, -20.96226629318544710 ) ) ;
#2799=CARTESIAN_POINT ( 'NONE',  ( 8.119414445536275338, 14.15357424190336566, 19.36786064314131650 ) ) ;
#2821=CARTESIAN_POINT ( 'NONE',  ( 8.484928971929276642, 14.69808267000900770, -19.21052728408403354 ) ) ;
#2826=CARTESIAN_POINT ( 'NONE',  ( -2.220931175283385350, 45.50830112210639555, 20.88445027029172962 ) ) ;
#2835=ORIENTED_EDGE ( 'NONE', *, *, #1174, .T. ) ;
#2839=PLANE ( 'NONE',  #8451 ) ;
#2843=CARTESIAN_POINT ( 'NONE',  ( 2.217630085887001279, 45.50684883240628409, -20.88476843860882326 ) ) ;
#2849=CARTESIAN_POINT ( 'NONE',  ( 8.654532730718658584, 25.02058024782134282, -23.45477484801500623 ) ) ;
#2879=ORIENTED_EDGE ( 'NONE', *, *, #11416, .F. ) ;
#2884=CARTESIAN_POINT ( 'NONE',  ( 9.478226885497544885, 16.74648819031018832, -18.74142151731972561 ) ) ;
#2906=CIRCLE ( 'NONE', #6153, 25.00000000000000000 ) ;
#2907=CARTESIAN_POINT ( 'NONE',  ( -3.307603021400832510, 53.76369073917810937, -20.73919124221722043 ) ) ;
#2937=CARTESIAN_POINT ( 'NONE',  ( 0.000000000000000000, 139.9999999999999716, 0.000000000000000000 ) ) ;
#2941=CARTESIAN_POINT ( 'NONE',  ( 4.337692624494786209, 47.49191884430658206, -24.62149689268095187 ) ) ;
#2972=CARTESIAN_POINT ( 'NONE',  ( -4.838792876751625727, 51.30218438880784504, 20.43503154247634868 ) ) ;
#2973=VECTOR ( 'NONE', #9723, 1000.000000000000000 ) ;
#2976=ORIENTED_EDGE ( 'NONE', *, *, #5725, .F. ) ;
#2977=EDGE_CURVE ( 'NONE', #1932, #1856, #573, .T. ) ;
#3003=CARTESIAN_POINT ( 'NONE',  ( 3.061616998149962604E-15, 10.00000000000000000, 25.00000000000000000 ) ) ;
#3017=CARTESIAN_POINT ( 'NONE',  ( 3.307338549894080604, 53.76391169785250668, -24.78134996739077422 ) ) ;
#3018=ORIENTED_EDGE ( 'NONE', *, *, #9369, .T. ) ;
#3030=CARTESIAN_POINT ( 'NONE',  ( 4.462445293788150025, 28.95508627606223229, 20.52252167446830100 ) ) ;
#3035=ORIENTED_EDGE ( 'NONE', *, *, #7930, .F. ) ;
#3036=CARTESIAN_POINT ( 'NONE',  ( -3.709758735690515970E-18, 30.00000000000001066, -25.00000000000000000 ) ) ;
#3067=CARTESIAN_POINT ( 'NONE',  ( 2.644456282953588921, 45.75339465611970269, -24.86012065554512063 ) ) ;
#3091=CARTESIAN_POINT ( 'NONE',  ( -0.8195736974120422236, 54.93507064933334050, 20.98461236856086032 ) ) ;
#3111=VERTEX_POINT ( 'NONE', #4133 ) ;
#3117=PRODUCT_DEFINITION_FORMATION_WITH_SPECIFIED_SOURCE ( 'ANY', '', #9041, .NOT_KNOWN. ) ;
#3129=CARTESIAN_POINT ( 'NONE',  ( 3.975724277407679974, 46.95046481276702366, -24.68253032026751370 ) ) ;
#3150=CARTESIAN_POINT ( 'NONE',  ( -8.118656623617184209, 14.15260872815194126, -19.36816941975095574 ) ) ;
#3152=CARTESIAN_POINT ( 'NONE',  ( 0.000000000000000000, 139.9999999999999716, 0.000000000000000000 ) ) ;
#3159=CARTESIAN_POINT ( 'NONE',  ( -1.612729787338046394, 45.25594143338945941, -24.94976830077123964 ) ) ;
#3160=CARTESIAN_POINT ( 'NONE',  ( -3.767196188295967918, 53.30371400289418915, 20.66066053404689029 ) ) ;
#3178=B_SPLINE_CURVE_WITH_KNOTS ( 'NONE', 3,
 ( #2509, #3464, #6561, #5501, #8288, #7520, #5560, #5374, #1678, #9370, #9245, #610, #12158, #11199, #7391, #10426, #11139, #1498, #3581, #670, #548, #4536, #6500, #4600, #7328, #3641 ),
 .UNSPECIFIED., .F., .F.,
 ( 4, 2, 2, 2, 2, 2, 2, 2, 2, 2, 2, 2, 4 ),
 ( 0.01580552869034228605, 0.01679261472842853362, 0.01777970076651477771, 0.01975387284268728671, 0.02172804491885978878, 0.02271513095694604328, 0.02370221699503229779, 0.02567638907120481373, 0.02666347510929107170, 0.02765056114737732967, 0.02962473322354984562, 0.03061181926163610706, 0.03159890529972236156 ),
 .UNSPECIFIED. ) ;
#3184=ORIENTED_EDGE ( 'NONE', *, *, #8798, .F. ) ;
#3185=CYLINDRICAL_SURFACE ( 'NONE', #325, 10.00000000000000355 ) ;
#3202=DIRECTION ( 'NONE',  ( -0.000000000000000000, -0.000000000000000000, 1.000000000000000000 ) ) ;
#3218=AXIS2_PLACEMENT_3D ( 'NONE', #5318, #9314, #373 ) ;
#3224=CARTESIAN_POINT ( 'NONE',  ( -4.968239015973206385, 50.65284130285913022, 20.40394647430411723 ) ) ;
#3226=VECTOR ( 'NONE', #2640, 1000.000000000000000 ) ;
#3228=CARTESIAN_POINT ( 'NONE',  ( 1.137587760790131908, 45.12834422743500085, 20.96978904175466596 ) ) ;
#3236=DIRECTION ( 'NONE',  ( 0.000000000000000000, 0.000000000000000000, 1.000000000000000000 ) ) ;
#3245=EDGE_CURVE ( 'NONE', #11306, #2044, #10375, .T. ) ;
#3255=CARTESIAN_POINT ( 'NONE',  ( -4.744071016079746350, 48.38731143956220393, 24.54607980264442091 ) ) ;
#3262=B_SPLINE_CURVE_WITH_KNOTS ( 'NONE', 3,
 ( #494, #4295, #6386, #4359, #2515, #11083, #4481, #3468, #8233, #3402, #6202, #11142, #7332, #5193, #3340, #5317, #1322, #9251, #7272, #6262, #4236, #2449, #6324, #8295, #10194, #2388 ),
 .UNSPECIFIED., .F., .F.,
 ( 4, 2, 2, 2, 2, 2, 2, 2, 2, 2, 2, 2, 4 ),
 ( 0.01580376012220196039, 0.01679085241551835084, 0.01777794470883474129, 0.01975212929546752219, 0.02172631388210030656, 0.02271340617541669701, 0.02370049846873308746, 0.02567468305536586837, 0.02666177534868225882, 0.02764886764199864927, 0.02962305222863143364, 0.03061014452194782409, 0.03159723681526421801 ),
 .UNSPECIFIED. ) ;
#3264=B_SPLINE_CURVE_WITH_KNOTS ( 'NONE', 3,
 ( #11410, #1948, #6583, #2778, #2720, #4685, #4619, #877, #2907, #4748, #8556, #6771, #8615, #10636, #11470, #4875, #3855, #12484, #3790, #10447 ),
 .UNSPECIFIED., .F., .F.,
 ( 4, 2, 2, 2, 2, 2, 2, 2, 2, 4 ),
 ( 3.491326639452381067E-19, 0.0009808062029949312765, 0.001961612405989862119, 0.002942418608984793179, 0.003923224811979723371, 0.004904031014974653997, 0.005884837217969585491, 0.006375240319467059477, 0.006865643420964533464, 0.007846449623959500519 ),
 .UNSPECIFIED. ) ;
#3278=ORIENTED_EDGE ( 'NONE', *, *, #4367, .T. ) ;
#3280=CARTESIAN_POINT ( 'NONE',  ( -8.651571107376318182, 25.02565239439968536, 23.45586713013333124 ) ) ;
#3286=CARTESIAN_POINT ( 'NONE',  ( 2.562745747226488176E-15, 30.00000000000001066, 21.00000000000000000 ) ) ;
#3289=CARTESIAN_POINT ( 'NONE',  ( 0.6529056306158902423, 45.03187583116404369, 20.99234021528525318 ) ) ;
#3313=VECTOR ( 'NONE', #946, 1000.000000000000000 ) ;
#3330=ORIENTED_EDGE ( 'NONE', *, *, #3811, .F. ) ;
#3337=CARTESIAN_POINT ( 'NONE',  ( -8.659888037695356644, 14.95771684574014948, -19.13532407230401944 ) ) ;
#3338=CARTESIAN_POINT ( 'NONE',  ( -2.619138840591237472, 29.67330545628644600, 24.87083797681799169 ) ) ;
#3340=CARTESIAN_POINT ( 'NONE',  ( -7.945999201647152788, 13.89399703635140249, 23.70671076423498391 ) ) ;
#3343=CARTESIAN_POINT ( 'NONE',  ( -6.197539731915355238E-14, 9.999999999999182876, 21.00000000000039080 ) ) ;
#3368=CARTESIAN_POINT ( 'NONE',  ( -6.197539731915355238E-14, 9.999999999999182876, 21.00000000000039080 ) ) ;
#3384=EDGE_CURVE ( 'NONE', #7013, #9272, #4628, .T. ) ;
#3398=CARTESIAN_POINT ( 'NONE',  ( 5.000000000000000000, 50.00000000000000000, 20.39607805437114152 ) ) ;
#3399=CARTESIAN_POINT ( 'NONE',  ( -6.109221465413982699, 27.94329460785578689, 24.24832107967536388 ) ) ;
#3401=EDGE_CURVE ( 'NONE', #11790, #4895, #2028, .T. ) ;
#3402=CARTESIAN_POINT ( 'NONE',  ( -5.845694806184612347, 11.88009017893230990, 24.30851799965319060 ) ) ;
#3404=CARTESIAN_POINT ( 'NONE',  ( -4.478749722781300235, 11.03480093803115558, 20.52614747825679942 ) ) ;
#3410=VERTEX_POINT ( 'NONE', #6511 ) ;
#3415=CARTESIAN_POINT ( 'NONE',  ( 0.6550203249928933102, 54.96765362015771927, 24.99347278016167095 ) ) ;
#3424=ORIENTED_EDGE ( 'NONE', *, *, #12017, .T. ) ;
#3433=EDGE_CURVE ( 'NONE', #10935, #2736, #5699, .T. ) ;
#3434=AXIS2_PLACEMENT_3D ( 'NONE', #5669, #12449, #9538 ) ;
#3440=CARTESIAN_POINT ( 'NONE',  ( -7.515231585295850891, 26.60501645963920225, 19.61046409729162932 ) ) ;
#3464=CARTESIAN_POINT ( 'NONE',  ( -10.00000000000000355, 19.66998333124466214, -22.91287847477919826 ) ) ;
#3465=CARTESIAN_POINT ( 'NONE',  ( -1.002883791299520887E-19, 10.00000000000000000, -25.00000000000000000 ) ) ;
#3468=CARTESIAN_POINT ( 'NONE',  ( -4.466051270639568749, 11.02833005318139925, 24.60558887372674519 ) ) ;
#3471=CYLINDRICAL_SURFACE ( 'NONE', #12424, 5.000000000000000000 ) ;
#3473=CARTESIAN_POINT ( 'NONE',  ( 5.303296350723960551, 28.48414319546200346, 24.43259468344301055 ) ) ;
#3476=CARTESIAN_POINT ( 'NONE',  ( 2.505975641493357831, 45.66085398937747186, 24.87560495202607669 ) ) ;
#3477=CARTESIAN_POINT ( 'NONE',  ( 3.971273688083300613, 53.05572982463418441, 24.68326415769028159 ) ) ;
#3494=CARTESIAN_POINT ( 'NONE',  ( -6.612279285637575832, 27.52949341102648262, 19.93770914801777749 ) ) ;
#3505=CARTESIAN_POINT ( 'NONE',  ( 10.00000000000000355, 20.00000000000000355, -28.00000000000000711 ) ) ;
#3512=CARTESIAN_POINT ( 'NONE',  ( 0.000000000000000000, 139.9999999999999716, -25.00000000000000000 ) ) ;
#3520=CARTESIAN_POINT ( 'NONE',  ( 1.648701702613829090, 10.13131270077370338, -24.94769321807935825 ) ) ;
#3526=CARTESIAN_POINT ( 'NONE',  ( -5.049704742916529376, 11.34434628041953452, 20.39145111578409697 ) ) ;
#3536=( GEOMETRIC_REPRESENTATION_CONTEXT ( 3 ) GLOBAL_UNCERTAINTY_ASSIGNED_CONTEXT ( ( #951 ) ) GLOBAL_UNIT_ASSIGNED_CONTEXT ( ( #4583, #1604, #3625 ) ) REPRESENTATION_CONTEXT ( 'NONE', 'WORKASPACE' ) );
#3543=CARTESIAN_POINT ( 'NONE',  ( -5.000000000000000000, 50.00000000000000000, -20.39607805437114152 ) ) ;
#3548=DIRECTION ( 'NONE',  ( -0.000000000000000000, -1.000000000000000000, -0.000000000000000000 ) ) ;
#3562=CARTESIAN_POINT ( 'NONE',  ( 2.295021694196371698, 10.26129700091049557, 20.87675788803829846 ) ) ;
#3572=DIRECTION ( 'NONE',  ( -0.000000000000000000, -0.000000000000000000, 1.000000000000000000 ) ) ;
#3576=CARTESIAN_POINT ( 'NONE',  ( 8.123360751522579193, 14.15902104166613107, 23.64419573351483450 ) ) ;
#3581=CARTESIAN_POINT ( 'NONE',  ( -4.146974088394097535, 10.89458658634673327, -24.65552811365946440 ) ) ;
#3589=DIRECTION ( 'NONE',  ( 0.000000000000000000, 1.000000000000000000, 0.000000000000000000 ) ) ;
#3593=CARTESIAN_POINT ( 'NONE',  ( -4.331872009808981794, 52.50234731214368367, 24.62196273622729592 ) ) ;
#3604=AXIS2_PLACEMENT_3D ( 'NONE', #9394, #10516, #7356 ) ;
#3618=CARTESIAN_POINT ( 'NONE',  ( -5.000000000000000000, 50.00000000000000000, 20.39607805437114152 ) ) ;
#3625=( NAMED_UNIT ( * ) SI_UNIT ( $, .STERADIAN. ) SOLID_ANGLE_UNIT ( ) );
#3627=ADVANCED_FACE ( 'NONE', ( #11184 ), #468, .F. ) ;
#3634=VERTEX_POINT ( 'NONE', #10114 ) ;
#3641=CARTESIAN_POINT ( 'NONE',  ( -1.002883791299520887E-19, 10.00000000000000000, -25.00000000000000000 ) ) ;
#3642=EDGE_CURVE ( 'NONE', #8125, #8822, #3658, .T. ) ;
#3658=CIRCLE ( 'NONE', #6307, 21.00000000000000000 ) ;
#3659=CARTESIAN_POINT ( 'NONE',  ( -9.657265040632822206, 22.61657440465215174, -18.64803156764659775 ) ) ;
#3660=DIRECTION ( 'NONE',  ( 0.000000000000000000, -0.000000000000000000, 1.000000000000000000 ) ) ;
#3668=CARTESIAN_POINT ( 'NONE',  ( 3.053082855025198494, 46.02690843307048141, -20.77868449535670692 ) ) ;
#3678=CARTESIAN_POINT ( 'NONE',  ( 0.000000000000000000, 50.00000000000000000, -28.00000000000000711 ) ) ;
#3686=CARTESIAN_POINT ( 'NONE',  ( -1.297374591076399408, 54.83977433137422253, -24.96837001061641104 ) ) ;
#3705=CARTESIAN_POINT ( 'NONE',  ( -4.493239192008157801, 47.78244187540930454, 20.51407495533472414 ) ) ;
#3730=EDGE_CURVE ( 'NONE', #5701, #7957, #9795, .T. ) ;
#3732=B_SPLINE_CURVE_WITH_KNOTS ( 'NONE', 3,
 ( #1993, #231, #1059, #8913, #5874, #4922, #104, #6940, #3964, #7965, #11833, #5409, #12132, #3440, #12254, #3494, #10223, #705, #11177, #5477, #6476, #9344, #10402, #9403, #646, #8980, #8031, #8446 ),
 .UNSPECIFIED., .F., .F.,
 ( 4, 2, 2, 2, 2, 2, 2, 2, 2, 2, 2, 2, 2, 4 ),
 ( 0.03175036704783668062, 0.03274152275842889814, 0.03373267846902110872, 0.03571498989020553683, 0.03670614560079775435, 0.03769730131138997187, 0.03868845702198218245, 0.03967961273257439997, 0.04166192415375883501, 0.04265307986435105253, 0.04364423557494327005, 0.04562654699612770509, 0.04661770270671992261, 0.04760885841731214013 ),
 .UNSPECIFIED. ) ;
#3757=CARTESIAN_POINT ( 'NONE',  ( -0.6685289520415670372, 30.00000000000001776, -25.00000000000001066 ) ) ;
#3766=CARTESIAN_POINT ( 'NONE',  ( -1.002883791299520887E-19, 10.00000000000000000, -25.00000000000000000 ) ) ;
#3771=CARTESIAN_POINT ( 'NONE',  ( -4.838567600861090057, 48.69772713945680209, 20.43508361496535031 ) ) ;
#3776=ORIENTED_EDGE ( 'NONE', *, *, #8676, .F. ) ;
#3782=CARTESIAN_POINT ( 'NONE',  ( -7.523626141222965025, 26.59539293290133344, -19.60723250985141775 ) ) ;
#3790=CARTESIAN_POINT ( 'NONE',  ( -4.999999999999999112, 50.32753737931852100, -20.39607805437113797 ) ) ;
#3795=CARTESIAN_POINT ( 'NONE',  ( 2.294321452706637121, 29.73876067080973229, -24.89658462890612967 ) ) ;
#3809=CARTESIAN_POINT ( 'NONE',  ( 6.843587254644259765, 12.70147400874256505, 19.85506230137591999 ) ) ;
#3811=EDGE_CURVE ( 'NONE', #3410, #7937, #11162, .T. ) ;
#3828=ORIENTED_EDGE ( 'NONE', *, *, #6489, .F. ) ;
#3855=CARTESIAN_POINT ( 'NONE',  ( -4.871666279273695999, 51.13754189277828743, -20.42713785987348984 ) ) ;
#3857=CARTESIAN_POINT ( 'NONE',  ( 9.918037823481203219, 21.32003297329905678, -18.51037319129331848 ) ) ;
#3880=LINE ( 'NONE', #10662, #1482 ) ;
#3885=DIRECTION ( 'NONE',  ( 0.000000000000000000, 1.000000000000000000, 0.000000000000000000 ) ) ;
#3892=ORIENTED_EDGE ( 'NONE', *, *, #5126, .F. ) ;
#3895=CARTESIAN_POINT ( 'NONE',  ( 0.000000000000000000, 20.00000000000000355, -28.00000000000000711 ) ) ;
#3918=CARTESIAN_POINT ( 'NONE',  ( -0.6578846949584694626, 54.95924935667866862, 20.99032885061396314 ) ) ;
#3950=FACE_OUTER_BOUND ( 'NONE', #9660, .T. ) ;
#3959=CYLINDRICAL_SURFACE ( 'NONE', #1967, 10.00000000000000355 ) ;
#3964=CARTESIAN_POINT ( 'NONE',  ( -8.955040573717580443, 24.46236383193878083, 18.99568595680172578 ) ) ;
#3968=CARTESIAN_POINT ( 'NONE',  ( 4.743537283058001819, 51.61420199850529400, -24.54618281552716041 ) ) ;
#3972=ORIENTED_EDGE ( 'NONE', *, *, #958, .T. ) ;
#4001=CARTESIAN_POINT ( 'NONE',  ( -3.050747483057216769, 53.97487283205587261, -24.81466456749452831 ) ) ;
#4008=CARTESIAN_POINT ( 'NONE',  ( -8.980220477185385519, 24.44733350940715866, -23.33298399582670157 ) ) ;
#4011=VERTEX_POINT ( 'NONE', #9273 ) ;
#4028=ORIENTED_EDGE ( 'NONE', *, *, #2398, .F. ) ;
#4041=CARTESIAN_POINT ( 'NONE',  ( -0.3266958997752330562, 45.00000000000001421, -25.00000000000000355 ) ) ;
#4042=CARTESIAN_POINT ( 'NONE',  ( -3.973286137925955863, 53.05282384735495782, 20.62152687101385951 ) ) ;
#4048=CARTESIAN_POINT ( 'NONE',  ( 5.034037828167091000, 28.66467738801596354, -24.49412005228846922 ) ) ;
#4098=CARTESIAN_POINT ( 'NONE',  ( -10.00000000000000355, 20.00000000000000355, -18.46618531261938401 ) ) ;
#4104=CARTESIAN_POINT ( 'NONE',  ( -4.484481976314367735, 47.78274414339135490, -24.59462526944309246 ) ) ;
#4132=CARTESIAN_POINT ( 'NONE',  ( -4.999999999999999112, 50.32713193883511593, -24.49489742783179125 ) ) ;
#4133=CARTESIAN_POINT ( 'NONE',  ( 5.340684424226280325E-17, 55.00000000000000000, -25.00000000000000000 ) ) ;
#4147=CARTESIAN_POINT ( 'NONE',  ( 2.222400765636041164, 54.49077458862202405, -20.88425590885463379 ) ) ;
#4161=EDGE_CURVE ( 'NONE', #11790, #9272, #9520, .T. ) ;
#4166=CARTESIAN_POINT ( 'NONE',  ( -9.983226034450831676, 19.33178880168245328, -18.47529793303663936 ) ) ;
#4175=EDGE_CURVE ( 'NONE', #5701, #3634, #6587, .T. ) ;
#4176=CARTESIAN_POINT ( 'NONE',  ( 1.342157722727130131E-15, 30.00000000000002132, -21.00000000000000355 ) ) ;
#4198=B_SPLINE_CURVE_WITH_KNOTS ( 'NONE', 3,
 ( #2078, #4819, #5008, #11671, #1144, #9705, #5898, #2147, #4941, #2849, #9896, #11733, #9643, #1020, #8745, #6776, #10642, #4048, #8807, #10834, #5773, #7926, #3795, #4881, #950, #11602, #8685, #3036 ),
 .UNSPECIFIED., .F., .F.,
 ( 4, 2, 2, 2, 2, 2, 2, 2, 2, 2, 2, 2, 2, 4 ),
 ( 0.04738924854463780201, 0.04936272659091893444, 0.05034946561405949372, 0.05133620463720005994, 0.05232294366034062616, 0.05330968268348119238, 0.05528316072976231788, 0.05626989975290288409, 0.05725663877604345031, 0.05923011682232458969, 0.06021685584546515591, 0.06120359486860571518, 0.06219033389174628140, 0.06317707291488684762 ),
 .UNSPECIFIED. ) ;
#4206=VECTOR ( 'NONE', #7834, 1000.000000000000000 ) ;
#4217=ADVANCED_FACE ( 'NONE', ( #1827 ), #6646, .F. ) ;
#4232=CARTESIAN_POINT ( 'NONE',  ( 10.00000000000000355, 20.00000000000000355, -22.91287847477919826 ) ) ;
#4236=CARTESIAN_POINT ( 'NONE',  ( -9.673562854105167474, 17.38029584746389133, 23.05303382818504332 ) ) ;
#4238=CARTESIAN_POINT ( 'NONE',  ( 6.119794236291119738, 27.93508701313207609, 20.09620109607250527 ) ) ;
#4251=CARTESIAN_POINT ( 'NONE',  ( 2.559760333650129958E-15, 55.00000000000000000, 21.00000000000000000 ) ) ;
#4270=ORIENTED_EDGE ( 'NONE', *, *, #6526, .F. ) ;
#4287=EDGE_CURVE ( 'NONE', #12540, #6613, #4198, .T. ) ;
#4290=CARTESIAN_POINT ( 'NONE',  ( -4.448741964560915640, 28.96190946584970405, 24.60274125495980613 ) ) ;
#4295=CARTESIAN_POINT ( 'NONE',  ( -0.3301927727158289749, 10.00000000000000000, 25.00000000000000355 ) ) ;
#4297=CARTESIAN_POINT ( 'NONE',  ( -7.945225341866328783, 13.89296426715405453, 19.44295823276161173 ) ) ;
#4299=CARTESIAN_POINT ( 'NONE',  ( 7.520704636030203893, 26.59870071877557507, -19.60835093631877513 ) ) ;
#4303=CARTESIAN_POINT ( 'NONE',  ( 3.052604782738682854, 46.02637368922790984, 24.81445626415020200 ) ) ;
#4337=B_SPLINE_CURVE_WITH_KNOTS ( 'NONE', 3,
 ( #8578, #2680, #775, #3686, #8891, #8007, #11808, #4001, #9849, #143, #2166, #8823, #6105, #8072, #10722, #7046, #4132, #6038 ),
 .UNSPECIFIED., .F., .F.,
 ( 4, 2, 2, 2, 2, 2, 2, 2, 4 ),
 ( 5.188175463412582976E-20, 0.0009797360301013575360, 0.001959472060202715072, 0.002939208090304072825, 0.003918944120405430144, 0.004898680150506787463, 0.005878416180608145650, 0.006858152210709502969, 0.007837888240810860288 ),
 .UNSPECIFIED. ) ;
#4344=VECTOR ( 'NONE', #3572, 1000.000000000000000 ) ;
#4352=DIRECTION ( 'NONE',  ( 0.000000000000000000, 0.000000000000000000, -1.000000000000000000 ) ) ;
#4355=CARTESIAN_POINT ( 'NONE',  ( 3.304769568038884664, 53.76613650905855479, 20.73964112051737274 ) ) ;
#4359=CARTESIAN_POINT ( 'NONE',  ( -1.325835098444672733, 10.08270123135439711, 24.96701611100131402 ) ) ;
#4364=CARTESIAN_POINT ( 'NONE',  ( 9.983143436873248788, 20.66859359106200955, 22.92025639428880623 ) ) ;
#4367=EDGE_CURVE ( 'NONE', #2044, #4011, #12050, .T. ) ;
#4369=CARTESIAN_POINT ( 'NONE',  ( 0.3299754220453550713, 55.00000000000001421, 25.00000000000000000 ) ) ;
#4389=CARTESIAN_POINT ( 'NONE',  ( -2.217326200926027724, 45.51555228448187762, 24.90189708455264395 ) ) ;
#4412=CARTESIAN_POINT ( 'NONE',  ( 7.537524037383855458, 13.39612119810769819, -23.84148986838564710 ) ) ;
#4418=CARTESIAN_POINT ( 'NONE',  ( -9.102716943808436767, 15.84719902056293250, 18.92511310367350319 ) ) ;
#4421=CARTESIAN_POINT ( 'NONE',  ( -2.221358530307614654, 54.49149874209361144, 24.90297606857491175 ) ) ;
#4454=CARTESIAN_POINT ( 'NONE',  ( -4.999999999999999112, 49.67330453822126657, 24.49489742783177348 ) ) ;
#4458=DIRECTION ( 'NONE',  ( -0.000000000000000000, -1.000000000000000000, -0.000000000000000000 ) ) ;
#4477=CARTESIAN_POINT ( 'NONE',  ( 3.246557057937244029, 10.51899376542992925, -24.79585947768713439 ) ) ;
#4481=CARTESIAN_POINT ( 'NONE',  ( -3.246935905771412667, 10.51876153604172970, 24.79592758899451255 ) ) ;
#4486=CARTESIAN_POINT ( 'NONE',  ( -4.246666789336575931, 52.64435674096336015, 24.63684932116156645 ) ) ;
#4488=CARTESIAN_POINT ( 'NONE',  ( 3.764226701178052803, 46.69296989397847852, 24.71608072572789538 ) ) ;
#4533=ORIENTED_EDGE ( 'NONE', *, *, #3245, .F. ) ;
#4536=CARTESIAN_POINT ( 'NONE',  ( -1.643512924178977430, 10.13039013404520716, -24.94805769307042453 ) ) ;
#4551=CARTESIAN_POINT ( 'NONE',  ( 1.298299055536097368, 45.16027954822755675, 24.96835849755778014 ) ) ;
#4560=DIRECTION ( 'NONE',  ( -0.000000000000000000, -1.000000000000000000, -0.000000000000000000 ) ) ;
#4583=( LENGTH_UNIT ( ) NAMED_UNIT ( * ) SI_UNIT ( .MILLI., .METRE. ) );
#4591=CARTESIAN_POINT ( 'NONE',  ( -2.290944097510326571, 29.73958545346254922, -24.89690719708686828 ) ) ;
#4600=CARTESIAN_POINT ( 'NONE',  ( -0.6576044892141179599, 10.01619439626406383, -24.99350884773162207 ) ) ;
#4605=CARTESIAN_POINT ( 'NONE',  ( -1.614219986190975620, 45.25635288715552207, 20.94008338602824182 ) ) ;
#4609=CARTESIAN_POINT ( 'NONE',  ( 9.737811142203947057, 22.29842083447240597, 23.02563804066124931 ) ) ;
#4611=ORIENTED_EDGE ( 'NONE', *, *, #100, .T. ) ;
#4619=CARTESIAN_POINT ( 'NONE',  ( -2.508870892452910173, 54.33730018467829126, -20.85139144392807253 ) ) ;
#4628=B_SPLINE_CURVE_WITH_KNOTS ( 'NONE', 3,
 ( #5512, #10438, #8483, #622, #2581, #9320, #7278, #3593, #4486, #11149, #5630, #12108, #9379, #10256, #4421, #558, #8361, #5447, #12354, #12292 ),
 .UNSPECIFIED., .F., .F.,
 ( 4, 2, 2, 2, 2, 2, 2, 2, 2, 4 ),
 ( 0.01567180661725443153, 0.01665134708417310289, 0.01763088755109177425, 0.01812065778455110993, 0.01861042801801044561, 0.01958996848492911697, 0.02056950895184778833, 0.02154904941876645622, 0.02252858988568512758, 0.02350813035260379893 ),
 .UNSPECIFIED. ) ;
#4629=VECTOR ( 'NONE', #2333, 1000.000000000000000 ) ;
#4638=CARTESIAN_POINT ( 'NONE',  ( -3.302322679538425287, 46.23143709543641933, -20.74005723812733848 ) ) ;
#4641=CARTESIAN_POINT ( 'NONE',  ( 7.297852186526522900, 13.15569421923598448, 19.69262651265845676 ) ) ;
#4646=CARTESIAN_POINT ( 'NONE',  ( 3.061616997868383043E-15, 0.000000000000000000, 25.00000000000000000 ) ) ;
#4652=B_SPLINE_CURVE_WITH_KNOTS ( 'NONE', 3,
 ( #769, #1776, #7624, #5660, #5723, #7498, #8509, #8573, #7370, #4638, #9408, #12259, #12384, #1600, #10465, #10406, #11487, #2675 ),
 .UNSPECIFIED., .F., .F.,
 ( 4, 2, 2, 2, 2, 2, 2, 2, 4 ),
 ( 0.007846449623959500519, 0.008826741871943226750, 0.009807034119926952981, 0.01078732636791067921, 0.01176761861589440544, 0.01274791086387813341, 0.01372820311186185790, 0.01470849535984558587, 0.01568878760782931384 ),
 .UNSPECIFIED. ) ;
#4653=LINE ( 'NONE', #10419, #4344 ) ;
#4681=CARTESIAN_POINT ( 'NONE',  ( -3.567510909640027705, 29.34773727012557387, -20.69703671296004188 ) ) ;
#4685=CARTESIAN_POINT ( 'NONE',  ( -2.222058947943490903, 54.49108331096404356, -20.88431890158240734 ) ) ;
#4718=( LENGTH_UNIT ( ) NAMED_UNIT ( * ) SI_UNIT ( .MILLI., .METRE. ) );
#4727=CIRCLE ( 'NONE', #12228, 25.00000000000000000 ) ;
#4732=DIRECTION ( 'NONE',  ( 0.000000000000000000, 0.000000000000000000, 1.000000000000000000 ) ) ;
#4741=B_SPLINE_CURVE_WITH_KNOTS ( 'NONE', 3,
 ( #5562, #924, #855, #7647, #1740, #11510, #10611, #2697, #7521, #7456, #8473, #11451, #794, #9371, #8657, #9555, #8594, #2821, #12526, #7709, #11577, #2884, #2636, #5502, #671, #6501, #1679, #9431 ),
 .UNSPECIFIED., .F., .F.,
 ( 4, 2, 2, 2, 2, 2, 2, 2, 2, 2, 2, 2, 2, 4 ),
 ( 0.03175360674246840986, 0.03274498614013845316, 0.03373636553780849645, 0.03571912433314858998, 0.03671050373081863327, 0.03770188312848867657, 0.03869326252615871986, 0.03968464192382877009, 0.04166740071916885668, 0.04265878011683889998, 0.04365015951450894327, 0.04563291830984904374, 0.04662429770751908703, 0.04761567710518913032 ),
 .UNSPECIFIED. ) ;
#4742=CARTESIAN_POINT ( 'NONE',  ( -2.301101458689752910, 29.73723473350772650, -20.87607290278878835 ) ) ;
#4748=CARTESIAN_POINT ( 'NONE',  ( -3.766953629715470431, 53.30388651120591703, -20.66069581306526004 ) ) ;
#4749=CARTESIAN_POINT ( 'NONE',  ( 3.024050948510435495E-21, 45.00000000000000711, -21.00000000000000000 ) ) ;
#4793=AXIS2_PLACEMENT_3D ( 'NONE', #3152, #10893, #6079 ) ;
#4803=UNCERTAINTY_MEASURE_WITH_UNIT (LENGTH_MEASURE( 1.000000000000000082E-05 ), #4718, 'distance_accuracy_value', 'NONE');
#4818=VERTEX_POINT ( 'NONE', #6676 ) ;
#4819=CARTESIAN_POINT ( 'NONE',  ( 10.00000000000000711, 20.65896320323604485, -22.91287847477919470 ) ) ;
#4836=ORIENTED_EDGE ( 'NONE', *, *, #3401, .T. ) ;
#4848=CARTESIAN_POINT ( 'NONE',  ( 5.022951428105686844, 11.32827475346531720, 24.49655794125914099 ) ) ;
#4862=CARTESIAN_POINT ( 'NONE',  ( 5.340684424226280325E-17, 55.00000000000000000, -25.00000000000000000 ) ) ;
#4867=CARTESIAN_POINT ( 'NONE',  ( -3.594513446512490388E-16, 55.00000000000000000, -21.00000000000000000 ) ) ;
#4870=CARTESIAN_POINT ( 'NONE',  ( -6.854073901798486190, 27.28868271418044245, -19.85144179826269450 ) ) ;
#4875=CARTESIAN_POINT ( 'NONE',  ( -4.831180326583886853, 51.29868641109617755, -20.43678301931617014 ) ) ;
#4877=CARTESIAN_POINT ( 'NONE',  ( 9.671223021026712274, 22.62837036926845968, -18.64106995571668079 ) ) ;
#4881=CARTESIAN_POINT ( 'NONE',  ( 1.651856453710261352, 29.86806670974593914, -24.94744891504881679 ) ) ;
#4895=VERTEX_POINT ( 'NONE', #3512 ) ;
#4912=CARTESIAN_POINT ( 'NONE',  ( 3.241086154805254083, 10.53405487867120982, 24.79105057270042067 ) ) ;
#4922=CARTESIAN_POINT ( 'NONE',  ( -9.670693212272151840, 22.62952413424389420, 18.64134173399714811 ) ) ;
#4924=ORIENTED_EDGE ( 'NONE', *, *, #6560, .T. ) ;
#4935=CARTESIAN_POINT ( 'NONE',  ( -4.967147891453746134, 49.34082981697670078, -24.50166768924217564 ) ) ;
#4941=CARTESIAN_POINT ( 'NONE',  ( 8.964356567778166252, 24.44381301785154292, -23.33811713236289620 ) ) ;
#4978=ORIENTED_EDGE ( 'NONE', *, *, #4161, .F. ) ;
#4992=EDGE_LOOP ( 'NONE', ( #3035, #9305, #5494, #5554, #1280, #11685 ) ) ;
#5004=CARTESIAN_POINT ( 'NONE',  ( 1.343687355773163672, 29.93123645385455944, -20.96702215260311064 ) ) ;
#5008=CARTESIAN_POINT ( 'NONE',  ( 9.935507569286025742, 21.31398369048515562, -22.94135581966985526 ) ) ;
#5023=ADVANCED_FACE ( 'NONE', ( #3950, #153 ), #7826, .T. ) ;
#5048=AXIS2_PLACEMENT_3D ( 'NONE', #2937, #3885, #7760 ) ;
#5056=CARTESIAN_POINT ( 'NONE',  ( -10.00000000000000355, 20.00000000000000355, -22.91287847477919826 ) ) ;
#5069=CARTESIAN_POINT ( 'NONE',  ( -4.329834338986901621, 47.49413952373966197, -24.62232128246942509 ) ) ;
#5070=CARTESIAN_POINT ( 'NONE',  ( -3.709758735690515970E-18, 30.00000000000001066, -25.00000000000000000 ) ) ;
#5102=CARTESIAN_POINT ( 'NONE',  ( 3.303834617765012194, 46.23291288788979614, -24.78182658752202983 ) ) ;
#5124=PRODUCT_DEFINITION ( 'UNKNOWN', '', #3117, #289 ) ;
#5125=CARTESIAN_POINT ( 'NONE',  ( -2.300052248552254319, 10.26239894176076994, -20.87624245596524730 ) ) ;
#5126=EDGE_CURVE ( 'NONE', #8822, #8125, #6455, .T. ) ;
#5152=VERTEX_POINT ( 'NONE', #9139 ) ;
#5156=VECTOR ( 'NONE', #8975, 1000.000000000000000 ) ;
#5158=DIRECTION ( 'NONE',  ( 1.000000000000000000, 0.000000000000000000, 0.000000000000000000 ) ) ;
#5183=CARTESIAN_POINT ( 'NONE',  ( 2.571758291765529985E-15, 45.00000000000000711, 21.00000000000000000 ) ) ;
#5189=CARTESIAN_POINT ( 'NONE',  ( -7.994063978020062912E-22, 10.00000000000000000, -21.00000000000000000 ) ) ;
#5193=CARTESIAN_POINT ( 'NONE',  ( -7.536850167683876833, 13.39586159374066021, 23.84162237519015548 ) ) ;
#5195=CARTESIAN_POINT ( 'NONE',  ( -0.6585108229100932187, 45.03273675766970285, -24.99339394906690970 ) ) ;
#5196=CARTESIAN_POINT ( 'NONE',  ( -4.336756015782423646, 52.50983733265497477, 20.54816100008359214 ) ) ;
#5198=CARTESIAN_POINT ( 'NONE',  ( 4.839481439987470601, 48.70147115714765107, 20.43486580129273733 ) ) ;
#5244=CYLINDRICAL_SURFACE ( 'NONE', #1593, 25.00000000000000000 ) ;
#5290=CARTESIAN_POINT ( 'NONE',  ( -4.838865259365938698, 48.69895664399926005, 24.52732495089485099 ) ) ;
#5292=DIRECTION ( 'NONE',  ( 0.000000000000000000, 1.000000000000000000, 0.000000000000000000 ) ) ;
#5314=CARTESIAN_POINT ( 'NONE',  ( -4.149932937002940747, 29.10413268181202184, 24.65505180927770112 ) ) ;
#5317=CARTESIAN_POINT ( 'NONE',  ( -8.488496443319393236, 14.70368316582932877, 23.51557330312556360 ) ) ;
#5318=CARTESIAN_POINT ( 'NONE',  ( 0.000000000000000000, 139.9999999999999716, 0.000000000000000000 ) ) ;
#5321=CARTESIAN_POINT ( 'NONE',  ( 9.867555937047535863, 21.65500574101911724, 22.97033549711487410 ) ) ;
#5322=CARTESIAN_POINT ( 'NONE',  ( 1.298746404259454534, 45.16883511797273343, 20.96039105888827692 ) ) ;
#5335=ORIENTED_EDGE ( 'NONE', *, *, #9402, .F. ) ;
#5351=CARTESIAN_POINT ( 'NONE',  ( -0.6591801397249409389, 45.03285316749953182, 24.99337097521990003 ) ) ;
#5353=CARTESIAN_POINT ( 'NONE',  ( 0.000000000000000000, 50.00000000000000000, -28.00000000000000711 ) ) ;
#5374=CARTESIAN_POINT ( 'NONE',  ( -8.972964902253410813, 15.53670184611763005, -23.33582545272828312 ) ) ;
#5375=CARTESIAN_POINT ( 'NONE',  ( 1.317448503741515342, 10.08163033484836113, -24.96744191981147409 ) ) ;
#5380=CYLINDRICAL_SURFACE ( 'NONE', #3218, 21.00000000000000000 ) ;
#5385=CARTESIAN_POINT ( 'NONE',  ( 0.6586899486374204749, 30.00000000000001421, 25.00000000000000000 ) ) ;
#5409=CARTESIAN_POINT ( 'NONE',  ( -8.119709436525981872, 25.84588397371641122, 19.36772275760405648 ) ) ;
#5414=CARTESIAN_POINT ( 'NONE',  ( -1.300905012451813336, 45.16112489716824996, 24.96819491493427634 ) ) ;
#5436=CARTESIAN_POINT ( 'NONE',  ( 2.559760333650129958E-15, 55.00000000000000000, 21.00000000000000000 ) ) ;
#5437=CARTESIAN_POINT ( 'NONE',  ( -9.673352204464322313, 22.61971715202064104, 23.05311956053869338 ) ) ;
#5447=CARTESIAN_POINT ( 'NONE',  ( -0.6582364880112170358, 54.96720335004231828, 24.99338302292539638 ) ) ;
#5452=B_SPLINE_CURVE_WITH_KNOTS ( 'NONE', 3,
 ( #5436, #12284, #2567, #5619, #11326, #731, #6383, #8472, #4355, #2635, #10190, #9430, #12342, #10248, #11387, #2696, #8227, #3398 ),
 .UNSPECIFIED., .F., .F.,
 ( 4, 2, 2, 2, 2, 2, 2, 2, 4 ),
 ( 0.02353265389067876051, 0.02451271468972987533, 0.02549277548878099361, 0.02647283628783211190, 0.02745289708688322672, 0.02843295788593434500, 0.02941301868498545982, 0.03039307948403657811, 0.03137314028308769293 ),
 .UNSPECIFIED. ) ;
#5453=CARTESIAN_POINT ( 'NONE',  ( 3.303926766530076442, 46.23304915065238418, 24.78181020466353601 ) ) ;
#5455=CARTESIAN_POINT ( 'NONE',  ( 4.838449599032471404, 51.30291823734444989, 24.52740775798701378 ) ) ;
#5477=CARTESIAN_POINT ( 'NONE',  ( -4.453030037920870932, 28.95979054136405395, 20.52457521359105996 ) ) ;
#5494=ORIENTED_EDGE ( 'NONE', *, *, #7004, .F. ) ;
#5501=CARTESIAN_POINT ( 'NONE',  ( -9.917336477930691174, 18.67442475474294028, -22.94880690262607459 ) ) ;
#5502=CARTESIAN_POINT ( 'NONE',  ( 9.867746314566257837, 18.34543089117788028, -18.53734326927642684 ) ) ;
#5506=FACE_OUTER_BOUND ( 'NONE', #141, .T. ) ;
#5507=CARTESIAN_POINT ( 'NONE',  ( -5.000000000000000000, 50.00000000000000000, 20.39607805437114152 ) ) ;
#5512=CARTESIAN_POINT ( 'NONE',  ( -5.000000000000000000, 50.00000000000000000, 24.49489742783178414 ) ) ;
#5528=ORIENTED_EDGE ( 'NONE', *, *, #6826, .F. ) ;
#5554=ORIENTED_EDGE ( 'NONE', *, *, #6489, .T. ) ;
#5560=CARTESIAN_POINT ( 'NONE',  ( -9.481501190889247255, 16.75403870714897536, -23.13387092261990574 ) ) ;
#5562=CARTESIAN_POINT ( 'NONE',  ( -7.994063978020062912E-22, 10.00000000000000000, -21.00000000000000000 ) ) ;
#5565=CARTESIAN_POINT ( 'NONE',  ( -2.511626000443172746, 45.66440847798708091, 20.85104232884582487 ) ) ;
#5570=CARTESIAN_POINT ( 'NONE',  ( 5.021458388981292487, 28.65403010179421983, 24.49227020900855933 ) ) ;
#5584=CARTESIAN_POINT ( 'NONE',  ( -10.00000000000000355, 20.00000000000000355, -28.00000000000000711 ) ) ;
#5587=ADVANCED_FACE ( 'NONE', ( #11204 ), #5380, .F. ) ;
#5591=CARTESIAN_POINT ( 'NONE',  ( 10.00000000000000355, 20.00000000000000355, -18.46618531261938401 ) ) ;
#5608=EDGE_CURVE ( 'NONE', #2364, #7013, #9123, .T. ) ;
#5615=CARTESIAN_POINT ( 'NONE',  ( 8.975091145622032585, 15.54177410167867990, 23.33498156074052687 ) ) ;
#5619=CARTESIAN_POINT ( 'NONE',  ( 1.296662627741595797, 54.84000786826194229, 20.96239067773004905 ) ) ;
#5630=CARTESIAN_POINT ( 'NONE',  ( -3.767201726441450571, 53.30370413573731980, 24.71563014075751141 ) ) ;
#5632=ORIENTED_EDGE ( 'NONE', *, *, #2201, .F. ) ;
#5641=CARTESIAN_POINT ( 'NONE',  ( 2.510026038814216598, 45.66334912595792161, -20.85125448412398441 ) ) ;
#5647=CARTESIAN_POINT ( 'NONE',  ( 10.00000000000000355, 20.00000000000000355, -28.00000000000000711 ) ) ;
#5660=CARTESIAN_POINT ( 'NONE',  ( -4.838593727670618350, 48.69800932989790709, -20.43507704550293624 ) ) ;
#5669=CARTESIAN_POINT ( 'NONE',  ( 0.000000000000000000, 0.000000000000000000, 0.000000000000000000 ) ) ;
#5699=B_SPLINE_CURVE_WITH_KNOTS ( 'NONE', 3,
 ( #866, #10566, #9987, #8020, #9565, #1940, #6117, #1002, #2769, #7723, #5817, #11589, #4147, #12476, #1297, #2181, #6053, #4867 ),
 .UNSPECIFIED., .F., .F.,
 ( 4, 2, 2, 2, 2, 2, 2, 2, 4 ),
 ( 0.02353287092482041556, 0.02451293455144068142, 0.02549299817806094728, 0.02647306180468121314, 0.02745312543130147553, 0.02843318905792174139, 0.02941325268454200725, 0.03039331631116227311, 0.03137337993778253897 ),
 .UNSPECIFIED. ) ;
#5701=VERTEX_POINT ( 'NONE', #7397 ) ;
#5704=FACE_BOUND ( 'NONE', #11894, .T. ) ;
#5723=CARTESIAN_POINT ( 'NONE',  ( -4.743665913102096177, 48.38584380519294825, -20.45762213685770092 ) ) ;
#5725=EDGE_CURVE ( 'NONE', #2044, #2364, #6931, .T. ) ;
#5726=B_SPLINE_CURVE_WITH_KNOTS ( 'NONE', 3,
 ( #6806, #11697, #8018, #5801, #7955, #1176, #7890, #9673, #3067, #281, #5102, #11821, #3129, #2941, #1109, #5926, #5865, #6996, #26, #10798 ),
 .UNSPECIFIED., .F., .F.,
 ( 4, 2, 2, 2, 2, 2, 2, 2, 2, 4 ),
 ( 0.01567185795944686308, 0.01665140573566027682, 0.01763095351187368709, 0.01812072739998039222, 0.01861050128808709736, 0.01959004906430051110, 0.02056959684051392484, 0.02154914461672733511, 0.02252869239294074538, 0.02350824016915415912 ),
 .UNSPECIFIED. ) ;
#5727=CARTESIAN_POINT ( 'NONE',  ( 8.970506128821204683, 15.53268569158106871, 18.98970815876138118 ) ) ;
#5762=CARTESIAN_POINT ( 'NONE',  ( -1.331065827029258131, 29.93295003906536067, -20.96783762878424895 ) ) ;
#5769=CARTESIAN_POINT ( 'NONE',  ( 5.000000000000000000, 50.00000000000000000, -28.00000000000000711 ) ) ;
#5770=CARTESIAN_POINT ( 'NONE',  ( 9.868178716563900110, 21.65205030131550146, -18.53711303768861640 ) ) ;
#5773=CARTESIAN_POINT ( 'NONE',  ( 3.238656815135313671, 29.46670881375417395, -24.79134413122120151 ) ) ;
#5774=SHAPE_DEFINITION_REPRESENTATION ( #226, #8235 ) ;
#5790=VECTOR ( 'NONE', #7087, 1000.000000000000000 ) ;
#5801=CARTESIAN_POINT ( 'NONE',  ( 1.300123024442352504, 45.16070347875686508, -24.96827571664099565 ) ) ;
#5805=LINE ( 'NONE', #9930, #4206 ) ;
#5812=EDGE_CURVE ( 'NONE', #4895, #3111, #2701, .T. ) ;
#5814=CARTESIAN_POINT ( 'NONE',  ( 0.3310707342383826801, 55.00000000000000711, -24.99999999999999645 ) ) ;
#5817=CARTESIAN_POINT ( 'NONE',  ( 3.054638161218191872, 53.97201501934328149, -20.77847170131455456 ) ) ;
#5823=CARTESIAN_POINT ( 'NONE',  ( -5.855196281420844251, 28.11311675345165995, -20.16916341828400761 ) ) ;
#5830=CARTESIAN_POINT ( 'NONE',  ( 9.983699295846122368, 20.66008309228626771, -18.47504095581592409 ) ) ;
#5848=CARTESIAN_POINT ( 'NONE',  ( 0.000000000000000000, 0.000000000000000000, 0.000000000000000000 ) ) ;
#5854=CARTESIAN_POINT ( 'NONE',  ( 0.000000000000000000, 139.9999999999999716, -21.00000000000000000 ) ) ;
#5857=DIRECTION ( 'NONE',  ( -0.000000000000000000, -0.000000000000000000, 1.000000000000000000 ) ) ;
#5865=CARTESIAN_POINT ( 'NONE',  ( 4.839602763736350788, 48.70207075804894714, -24.52717836283222752 ) ) ;
#5873=DIRECTION ( 'NONE',  ( -0.000000000000000000, -0.000000000000000000, 1.000000000000000000 ) ) ;
#5874=CARTESIAN_POINT ( 'NONE',  ( -9.867139490978726002, 21.65793074649777594, 18.53766545382552167 ) ) ;
#5877=CARTESIAN_POINT ( 'NONE',  ( 3.651743720672741667, 53.41923203171982237, -24.73212923346887848 ) ) ;
#5888=DIRECTION ( 'NONE',  ( 0.000000000000000000, 1.000000000000000000, 0.000000000000000000 ) ) ;
#5891=CARTESIAN_POINT ( 'NONE',  ( 10.00000000000000355, 20.67071788932440413, 18.46618531261938756 ) ) ;
#5892=CARTESIAN_POINT ( 'NONE',  ( -4.743108530676050982, 51.61529827254528158, 20.45774488160513371 ) ) ;
#5896=ORIENTED_EDGE ( 'NONE', *, *, #9071, .T. ) ;
#5898=CARTESIAN_POINT ( 'NONE',  ( 9.355409448593292154, 23.54720254436722371, -23.18392859692124830 ) ) ;
#5907=EDGE_CURVE ( 'NONE', #2444, #4011, #3732, .T. ) ;
#5922=CARTESIAN_POINT ( 'NONE',  ( -9.935193375007562722, 21.31442233758455274, -22.94148538850174646 ) ) ;
#5924=ORIENTED_EDGE ( 'NONE', *, *, #10368, .F. ) ;
#5926=CARTESIAN_POINT ( 'NONE',  ( 4.743618752923510762, 48.38567045510036735, -24.54617134760821173 ) ) ;
#5940=ORIENTED_EDGE ( 'NONE', *, *, #7973, .T. ) ;
#5941=CARTESIAN_POINT ( 'NONE',  ( 0.000000000000000000, 20.00000000000000355, -28.00000000000000711 ) ) ;
#5944=VECTOR ( 'NONE', #9309, 1000.000000000000000 ) ;
#5951=CARTESIAN_POINT ( 'NONE',  ( 1.342157722727130131E-15, 30.00000000000002132, -21.00000000000000355 ) ) ;
#5952=CARTESIAN_POINT ( 'NONE',  ( 4.743517746076369335, 48.38525476062307717, -20.45765889729212716 ) ) ;
#5963=DIRECTION ( 'NONE',  ( 0.000000000000000000, 1.000000000000000000, 0.000000000000000000 ) ) ;
#5970=CARTESIAN_POINT ( 'NONE',  ( -10.00000000000000355, 20.00000000000000355, -18.46618531261938401 ) ) ;
#5971=ORIENTED_EDGE ( 'NONE', *, *, #3642, .F. ) ;
#5978=B_SPLINE_CURVE_WITH_KNOTS ( 'NONE', 3,
 ( #1071, #11980, #4935, #9826, #8803, #8048, #4104, #5069, #8934, #11916, #120, #7085, #1324, #2274, #7983, #3159, #8867, #5195, #4041, #10016 ),
 .UNSPECIFIED., .F., .F.,
 ( 4, 2, 2, 2, 2, 2, 2, 2, 2, 4 ),
 ( 0.007837888240810860288, 0.008817134455640363022, 0.009796380670469867491, 0.01028600377788460932, 0.01077562688529935114, 0.01175487310012885388, 0.01273411931495835661, 0.01371336552978785761, 0.01469261174461736208, 0.01567185795944686308 ),
 .UNSPECIFIED. ) ;
#6004=CARTESIAN_POINT ( 'NONE',  ( 4.493076325134499172, 52.21789521489533570, -24.59326131088672440 ) ) ;
#6010=CARTESIAN_POINT ( 'NONE',  ( -10.00000000000000178, 19.66809010557521020, -18.46618531261939111 ) ) ;
#6015=CARTESIAN_POINT ( 'NONE',  ( 3.257619892980143650, 29.47720406012850347, 20.75490610440258621 ) ) ;
#6020=CARTESIAN_POINT ( 'NONE',  ( 0.3275525315169112162, 44.99999999999999289, 20.99999999999999645 ) ) ;
#6038=CARTESIAN_POINT ( 'NONE',  ( -5.000000000000000000, 50.00000000000000000, -24.49489742783178059 ) ) ;
#6042=ADVANCED_FACE ( 'NONE', ( #9528 ), #8629, .F. ) ;
#6046=CARTESIAN_POINT ( 'NONE',  ( -6.610481451048220158, 27.51047402958706201, -24.11159121895188306 ) ) ;
#6053=CARTESIAN_POINT ( 'NONE',  ( 0.3314803829344796782, 55.00000000000000000, -21.00000000000000000 ) ) ;
#6069=CARTESIAN_POINT ( 'NONE',  ( 1.302929565828678582, 54.83844695853547790, -24.96811105270434439 ) ) ;
#6079=DIRECTION ( 'NONE',  ( 0.000000000000000000, 0.000000000000000000, -1.000000000000000000 ) ) ;
#6083=CARTESIAN_POINT ( 'NONE',  ( 6.619094116331253552, 27.52385718499909117, 19.93550969653868066 ) ) ;
#6084=CARTESIAN_POINT ( 'NONE',  ( -5.000000000000000000, 50.00000000000000000, 20.39607805437114152 ) ) ;
#6105=CARTESIAN_POINT ( 'NONE',  ( -4.493909509445460415, 52.21603442804438799, -24.59310644668742540 ) ) ;
#6115=CARTESIAN_POINT ( 'NONE',  ( -3.768871583585197360, 46.69794849765531808, 24.71539284385418611 ) ) ;
#6117=CARTESIAN_POINT ( 'NONE',  ( 4.339277897004357953, 52.50559309311499590, -20.54763125150147829 ) ) ;
#6118=VERTEX_POINT ( 'NONE', #4251 ) ;
#6119=B_SPLINE_CURVE_WITH_KNOTS ( 'NONE', 3,
 ( #3465, #6441, #7140, #5375, #3520, #611, #4477, #8104, #11017, #11140, #10305, #8167, #550, #4412, #8289, #1565, #7329, #9182, #1621, #8228, #9058, #11972, #489, #7267, #369, #4232 ),
 .UNSPECIFIED., .F., .F.,
 ( 4, 2, 2, 2, 2, 2, 2, 2, 2, 2, 2, 2, 4 ),
 ( 0.03159890529972236156, 0.03258580175252957789, 0.03357269820533679422, 0.03554649111095121994, 0.03653338756375844321, 0.03752028401656565260, 0.03949407692218008525, 0.04146786982779451791, 0.04245476628060172730, 0.04344166273340894363, 0.04541545563902336935, 0.04640235209183058568, 0.04738924854463780201 ),
 .UNSPECIFIED. ) ;
#6135=EDGE_LOOP ( 'NONE', ( #10232, #6661, #12396, #4924, #3828, #5632 ) ) ;
#6136=CARTESIAN_POINT ( 'NONE',  ( -1.319698576403261825, 10.06506897208606333, -20.96877090753543627 ) ) ;
#6141=CARTESIAN_POINT ( 'NONE',  ( 1.321325188649778548, 29.91787852503522771, 20.96099891843594065 ) ) ;
#6142=CARTESIAN_POINT ( 'NONE',  ( -0.1649528864959406427, 55.00000000000000000, 21.00000000000000355 ) ) ;
#6151=CARTESIAN_POINT ( 'NONE',  ( 4.491430111798321967, 52.22103771687890372, 24.59356092490497758 ) ) ;
#6153=AXIS2_PLACEMENT_3D ( 'NONE', #677, #3589, #4732 ) ;
#6195=CARTESIAN_POINT ( 'NONE',  ( -7.300087775502666965, 26.84214942138161675, 23.91163959704068631 ) ) ;
#6196=LINE ( 'NONE', #10192, #5944 ) ;
#6202=CARTESIAN_POINT ( 'NONE',  ( -6.106142575418606278, 12.07400325324896784, 24.24423224237354901 ) ) ;
#6204=CARTESIAN_POINT ( 'NONE',  ( -10.00000000000000355, 20.00000000000000355, 18.46618531261938756 ) ) ;
#6205=DIRECTION ( 'NONE',  ( 0.000000000000000000, 0.000000000000000000, 1.000000000000000000 ) ) ;
#6239=DIRECTION ( 'NONE',  ( -0.000000000000000000, -0.000000000000000000, 1.000000000000000000 ) ) ;
#6253=FACE_OUTER_BOUND ( 'NONE', #2124, .T. ) ;
#6257=CARTESIAN_POINT ( 'NONE',  ( -8.123193803314322281, 25.84109844632562769, 23.64424386314666648 ) ) ;
#6262=CARTESIAN_POINT ( 'NONE',  ( -9.481487189274945493, 16.75591109918640242, 23.13382230614692148 ) ) ;
#6263=CARTESIAN_POINT ( 'NONE',  ( -5.000000000000000000, 50.00000000000000000, -28.00000000000000711 ) ) ;
#6268=CARTESIAN_POINT ( 'NONE',  ( 6.611279324052055095, 27.53068265742442122, 24.11471400905219298 ) ) ;
#6292=CARTESIAN_POINT ( 'NONE',  ( 0.000000000000000000, 139.9999999999999716, -21.00000000000000000 ) ) ;
#6307=AXIS2_PLACEMENT_3D ( 'NONE', #7373, #5292, #1480 ) ;
#6318=ORIENTED_EDGE ( 'NONE', *, *, #6668, .T. ) ;
#6324=CARTESIAN_POINT ( 'NONE',  ( -9.918789871757258680, 18.68607266337350836, 22.94817778295035993 ) ) ;
#6328=CARTESIAN_POINT ( 'NONE',  ( 4.149575074854375600, 29.10425525072577102, 24.65509887497819008 ) ) ;
#6332=B_SPLINE_CURVE_WITH_KNOTS ( 'NONE', 3,
 ( #7246, #9223, #5351, #5414, #2424, #529, #4389, #12136, #10996, #2484, #2248, #6115, #11059, #8267, #7122, #3255, #5290, #7182, #4454, #2306 ),
 .UNSPECIFIED., .F., .F.,
 ( 4, 2, 2, 2, 2, 2, 2, 2, 2, 4 ),
 ( 0.007837842730401771429, 0.008817088216258357411, 0.009796333702114945127, 0.01028595644504323552, 0.01077557918797152590, 0.01175482467382810668, 0.01273407015968468919, 0.01371331564554126997, 0.01469256113139785075, 0.01567180661725443153 ),
 .UNSPECIFIED. ) ;
#6333=CARTESIAN_POINT ( 'NONE',  ( 1.614504882520976681, 45.25664461204844713, 24.94963714481321304 ) ) ;
#6335=CARTESIAN_POINT ( 'NONE',  ( 2.217963917954424602, 54.49304390046189894, 24.90325875173717662 ) ) ;
#6383=CARTESIAN_POINT ( 'NONE',  ( 2.505765861943965334, 54.33918026639940990, 20.85177847850087574 ) ) ;
#6384=CARTESIAN_POINT ( 'NONE',  ( -7.930305867179300527, 26.10041404063223780, 23.70984975861344779 ) ) ;
#6386=CARTESIAN_POINT ( 'NONE',  ( -0.6638428588095105498, 10.01651532611708895, 24.99338002059894137 ) ) ;
#6390=CARTESIAN_POINT ( 'NONE',  ( 0.000000000000000000, 50.00000000000000000, -28.00000000000000711 ) ) ;
#6406=ORIENTED_EDGE ( 'NONE', *, *, #7973, .F. ) ;
#6408=DIRECTION ( 'NONE',  ( -0.000000000000000000, -0.000000000000000000, 1.000000000000000000 ) ) ;
#6441=CARTESIAN_POINT ( 'NONE',  ( 0.3289161358670515400, 10.00000000000000355, -25.00000000000000711 ) ) ;
#6447=CARTESIAN_POINT ( 'NONE',  ( -9.655964325742520060, 17.37895558718825129, 18.64870055153495798 ) ) ;
#6448=DIRECTION ( 'NONE',  ( 0.000000000000000000, 1.000000000000000000, 0.000000000000000000 ) ) ;
#6450=CARTESIAN_POINT ( 'NONE',  ( 6.112888882359681197, 27.94072674827362590, 24.24745615746033423 ) ) ;
#6455=CIRCLE ( 'NONE', #384, 21.00000000000000000 ) ;
#6463=CARTESIAN_POINT ( 'NONE',  ( -10.00000000000000355, 20.00000000000000355, 22.91287847477919826 ) ) ;
#6476=CARTESIAN_POINT ( 'NONE',  ( -4.158531974891625183, 29.10015071429011613, 20.58640575284740493 ) ) ;
#6489=EDGE_CURVE ( 'NONE', #10467, #10935, #9700, .T. ) ;
#6500=CARTESIAN_POINT ( 'NONE',  ( -1.314141907159803946, 10.08123752450589095, -24.96759818712484957 ) ) ;
#6501=CARTESIAN_POINT ( 'NONE',  ( 9.983665930786834508, 19.33914921762187689, -18.47505920260298851 ) ) ;
#6510=CARTESIAN_POINT ( 'NONE',  ( 8.124594680848492345, 25.83911103074633075, 23.64375881965231230 ) ) ;
#6511=CARTESIAN_POINT ( 'NONE',  ( 0.000000000000000000, 0.000000000000000000, -21.00000000000000000 ) ) ;
#6515=CARTESIAN_POINT ( 'NONE',  ( 5.000000000000000000, 50.00000000000000000, 24.49489742783178059 ) ) ;
#6520=CARTESIAN_POINT ( 'NONE',  ( -9.868806730738530320, 21.64797418619996350, 22.96979908047426377 ) ) ;
#6526=EDGE_CURVE ( 'NONE', #9164, #9118, #10512, .T. ) ;
#6536=ORIENTED_EDGE ( 'NONE', *, *, #7004, .T. ) ;
#6540=CARTESIAN_POINT ( 'NONE',  ( 6.605462518297898100, 12.48519332047425578, 19.93580698149260400 ) ) ;
#6556=CARTESIAN_POINT ( 'NONE',  ( 9.659257073854845999, 17.39080730681331488, 23.05883108104414347 ) ) ;
#6560=EDGE_CURVE ( 'NONE', #2695, #10935, #1266, .T. ) ;
#6561=CARTESIAN_POINT ( 'NONE',  ( -9.983516779091171855, 19.33659569722678029, -22.92009366892111899 ) ) ;
#6576=CARTESIAN_POINT ( 'NONE',  ( -9.351975853621407708, 23.55614770899448374, -18.80319155380984242 ) ) ;
#6583=CARTESIAN_POINT ( 'NONE',  ( -0.6576844598599284053, 54.96731546091645271, -20.99214996227340180 ) ) ;
#6587=LINE ( 'NONE', #5647, #1455 ) ;
#6600=ORIENTED_EDGE ( 'NONE', *, *, #11811, .F. ) ;
#6611=CARTESIAN_POINT ( 'NONE',  ( -1.324565580760808992, 29.93364609169914914, -24.97324923543901320 ) ) ;
#6613=VERTEX_POINT ( 'NONE', #5070 ) ;
#6624=CARTESIAN_POINT ( 'NONE',  ( -0.6600009463833134138, 45.03295123165366931, 20.99208596347618538 ) ) ;
#6646=CYLINDRICAL_SURFACE ( 'NONE', #3604, 5.000000000000000000 ) ;
#6661=ORIENTED_EDGE ( 'NONE', *, *, #7930, .T. ) ;
#6663=CARTESIAN_POINT ( 'NONE',  ( 9.462075664854227242, 16.74749304780872450, 18.74782784431838323 ) ) ;
#6668=EDGE_CURVE ( 'NONE', #2364, #6118, #10945, .T. ) ;
#6676=CARTESIAN_POINT ( 'NONE',  ( 0.000000000000000000, 0.000000000000000000, -25.00000000000000000 ) ) ;
#6690=CARTESIAN_POINT ( 'NONE',  ( -4.967254743859118804, 49.34118944982712662, 20.40418484253504516 ) ) ;
#6702=CARTESIAN_POINT ( 'NONE',  ( -8.127963825975040635, 25.83452922977894772, -19.36426980763129180 ) ) ;
#6707=CARTESIAN_POINT ( 'NONE',  ( 0.6528672473846522939, 45.03176223275875856, -20.99236587649955865 ) ) ;
#6712=ADVANCED_FACE ( 'NONE', ( #10310 ), #3471, .F. ) ;
#6771=CARTESIAN_POINT ( 'NONE',  ( -4.338943459110875089, 52.50631594060026686, -20.54770844439775956 ) ) ;
#6773=CARTESIAN_POINT ( 'NONE',  ( 8.957954983704073726, 24.45660132507920537, -18.99431620520108766 ) ) ;
#6776=CARTESIAN_POINT ( 'NONE',  ( 6.099398173400666145, 27.93114403207803420, -24.24592268179950594 ) ) ;
#6806=CARTESIAN_POINT ( 'NONE',  ( 6.955575927950914131E-22, 45.00000000000000711, -25.00000000000000000 ) ) ;
#6824=ORIENTED_EDGE ( 'NONE', *, *, #2977, .F. ) ;
#6826=EDGE_CURVE ( 'NONE', #9118, #4818, #4727, .T. ) ;
#6829=AXIS2_PLACEMENT_3D ( 'NONE', #2007, #5888, #1199 ) ;
#6831=CARTESIAN_POINT ( 'NONE',  ( -9.463424455697749593, 23.24851154398614739, -18.74714503555872724 ) ) ;
#6869=ORIENTED_EDGE ( 'NONE', *, *, #11969, .T. ) ;
#6871=CARTESIAN_POINT ( 'NONE',  ( 0.6608155348566246978, 10.00000000000000178, 24.99999999999999645 ) ) ;
#6883=CARTESIAN_POINT ( 'NONE',  ( 2.508429781980343609, 54.33777489521010295, -24.87536199211671573 ) ) ;
#6895=CARTESIAN_POINT ( 'NONE',  ( 9.099320553259442335, 24.16039445067871583, 18.92675418898895501 ) ) ;
#6896=CARTESIAN_POINT ( 'NONE',  ( 4.959250951056511703, 49.34212978433561858, -20.40603120131224557 ) ) ;
#6909=VECTOR ( 'NONE', #3548, 1000.000000000000000 ) ;
#6919=EDGE_CURVE ( 'NONE', #4895, #11790, #2906, .T. ) ;
#6925=CARTESIAN_POINT ( 'NONE',  ( -7.946065455725393356, 26.10639172058064972, -23.70672747870507280 ) ) ;
#6929=CARTESIAN_POINT ( 'NONE',  ( 3.548862490157215444, 10.64523530928737749, 24.74869899623665503 ) ) ;
#6931=B_SPLINE_CURVE_WITH_KNOTS ( 'NONE', 3,
 ( #10370, #1683, #6624, #10432, #4605, #2826, #5565, #12408, #859, #10495, #9621, #11455, #3705, #9558, #3771, #6690, #2574, #5507 ),
 .UNSPECIFIED., .F., .F.,
 ( 4, 2, 2, 2, 2, 2, 2, 2, 4 ),
 ( 0.007846355738354819295, 0.008826646719051039688, 0.009806937699747258347, 0.01078722868044347874, 0.01176751966113969913, 0.01274781064183591779, 0.01372810162253213818, 0.01470839260322835684, 0.01568868358392457724 ),
 .UNSPECIFIED. ) ;
#6940=CARTESIAN_POINT ( 'NONE',  ( -9.096797777268143648, 24.16610281865074583, 18.92797567942162829 ) ) ;
#6944=CARTESIAN_POINT ( 'NONE',  ( 3.968701803879573831, 53.04568146648268367, -24.68320166897649770 ) ) ;
#6946=ORIENTED_EDGE ( 'NONE', *, *, #5725, .T. ) ;
#6963=CARTESIAN_POINT ( 'NONE',  ( 4.337416167900176589, 47.49133373970335015, 20.54801971059908894 ) ) ;
#6996=CARTESIAN_POINT ( 'NONE',  ( 4.967203680380478659, 49.34177296812513447, -24.50165547367289065 ) ) ;
#7004=EDGE_CURVE ( 'NONE', #10467, #3111, #2466, .T. ) ;
#7013=VERTEX_POINT ( 'NONE', #42 ) ;
#7025=CARTESIAN_POINT ( 'NONE',  ( -3.306282206746268937, 53.76494240372728939, 20.73941076293121810 ) ) ;
#7046=CARTESIAN_POINT ( 'NONE',  ( -4.968205859249467338, 50.65222807605660904, -24.50145347565533882 ) ) ;
#7068=EDGE_CURVE ( 'NONE', #7957, #7937, #6196, .T. ) ;
#7073=CARTESIAN_POINT ( 'NONE',  ( 1.620000493755592075, 54.74147302055352071, -24.94927790585931504 ) ) ;
#7085=CARTESIAN_POINT ( 'NONE',  ( -3.302172444309792620, 46.23123523635531740, -24.78206517003335208 ) ) ;
#7086=CARTESIAN_POINT ( 'NONE',  ( -3.050155127176687575, 53.97520719309672188, 20.77909757380590250 ) ) ;
#7087=DIRECTION ( 'NONE',  ( -0.000000000000000000, -1.000000000000000000, -0.000000000000000000 ) ) ;
#7122=CARTESIAN_POINT ( 'NONE',  ( -4.493559251511619834, 47.78304274923282691, 24.59317321405577772 ) ) ;
#7128=CARTESIAN_POINT ( 'NONE',  ( -7.994063978020062912E-22, 10.00000000000000000, -21.00000000000000000 ) ) ;
#7140=CARTESIAN_POINT ( 'NONE',  ( 0.6581862696184550554, 10.01618719080246578, -24.99351150626209161 ) ) ;
#7154=DIRECTION ( 'NONE',  ( -0.000000000000000000, -1.000000000000000000, -0.000000000000000000 ) ) ;
#7157=VECTOR ( 'NONE', #9453, 1000.000000000000000 ) ;
#7174=CARTESIAN_POINT ( 'NONE',  ( -5.000000000000000000, 50.00000000000000000, -24.49489742783178059 ) ) ;
#7182=CARTESIAN_POINT ( 'NONE',  ( -4.967261190099589108, 49.34148114543111774, 24.50164489405593571 ) ) ;
#7201=CARTESIAN_POINT ( 'NONE',  ( -7.511663825336949429, 13.39091019075763533, -19.61183490434176235 ) ) ;
#7202=CARTESIAN_POINT ( 'NONE',  ( -0.6600000499078774174, 29.98375368882421910, 24.99348755773349140 ) ) ;
#7211=CARTESIAN_POINT ( 'NONE',  ( -2.625488409636790088, 10.34519051174632764, 20.83765690359550860 ) ) ;
#7212=DIRECTION ( 'NONE',  ( -0.000000000000000000, -0.000000000000000000, 1.000000000000000000 ) ) ;
#7213=CARTESIAN_POINT ( 'NONE',  ( 3.061617454482527662E-15, 30.00000000000001066, 25.00000000000000000 ) ) ;
#7215=ORIENTED_EDGE ( 'NONE', *, *, #985, .T. ) ;
#7220=CARTESIAN_POINT ( 'NONE',  ( 4.967390183827647299, 49.34301876381886132, 24.50161767623307441 ) ) ;
#7228=CARTESIAN_POINT ( 'NONE',  ( 3.061616997868383043E-15, 139.9999999999999716, 25.00000000000000000 ) ) ;
#7233=ORIENTED_EDGE ( 'NONE', *, *, #10024, .T. ) ;
#7246=CARTESIAN_POINT ( 'NONE',  ( 3.061617023331388775E-15, 45.00000000000000711, 25.00000000000000000 ) ) ;
#7267=CARTESIAN_POINT ( 'NONE',  ( 9.983753628317437290, 19.33993981085001579, -22.91999041428549688 ) ) ;
#7272=CARTESIAN_POINT ( 'NONE',  ( -9.106574839427329593, 15.85560948713796492, 23.28279145951148266 ) ) ;
#7278=CARTESIAN_POINT ( 'NONE',  ( -4.486434092443181143, 52.21331568334087336, 24.59426911350885092 ) ) ;
#7284=CARTESIAN_POINT ( 'NONE',  ( 1.295572856795887295, 54.84026084924703071, 24.96846459459551681 ) ) ;
#7291=ORIENTED_EDGE ( 'NONE', *, *, #7068, .T. ) ;
#7294=( GEOMETRIC_REPRESENTATION_CONTEXT ( 3 ) GLOBAL_UNCERTAINTY_ASSIGNED_CONTEXT ( ( #4803 ) ) GLOBAL_UNIT_ASSIGNED_CONTEXT ( ( #4718, #10299, #666 ) ) REPRESENTATION_CONTEXT ( 'NONE', 'WORKASPACE' ) );
#7322=ORIENTED_EDGE ( 'NONE', *, *, #5608, .T. ) ;
#7327=ORIENTED_EDGE ( 'NONE', *, *, #5126, .T. ) ;
#7328=CARTESIAN_POINT ( 'NONE',  ( -0.3289793214801078336, 10.00000000000000000, -25.00000000000000355 ) ) ;
#7329=CARTESIAN_POINT ( 'NONE',  ( 8.653999659896598473, 14.97853430653165319, -23.45497003317995421 ) ) ;
#7332=CARTESIAN_POINT ( 'NONE',  ( -6.851336394414588860, 12.70864359358585460, 24.04404201862471524 ) ) ;
#7336=CARTESIAN_POINT ( 'NONE',  ( -1.659969451079500224, 10.13322420983673311, 20.93680794575981352 ) ) ;
#7338=CARTESIAN_POINT ( 'NONE',  ( 5.000000000000000000, 50.00000000000000000, 24.49489742783178059 ) ) ;
#7341=EDGE_CURVE ( 'NONE', #2752, #6613, #2186, .T. ) ;
#7342=CARTESIAN_POINT ( 'NONE',  ( 5.000000000000000000, 50.00000000000000000, 24.49489742783178059 ) ) ;
#7356=DIRECTION ( 'NONE',  ( 1.000000000000000000, 0.000000000000000000, 0.000000000000000000 ) ) ;
#7370=CARTESIAN_POINT ( 'NONE',  ( -3.765972656198162571, 46.69472370319601850, -20.66089928520440111 ) ) ;
#7373=CARTESIAN_POINT ( 'NONE',  ( 0.000000000000000000, 139.9999999999999716, 0.000000000000000000 ) ) ;
#7391=CARTESIAN_POINT ( 'NONE',  ( -6.110563603929655585, 12.05744620208248286, -24.24805373538051967 ) ) ;
#7397=CARTESIAN_POINT ( 'NONE',  ( 10.00000000000000355, 20.00000000000000355, 18.46618531261938401 ) ) ;
#7399=CARTESIAN_POINT ( 'NONE',  ( -8.656678912164643691, 14.98331879925162902, 19.13349105540200057 ) ) ;
#7409=CARTESIAN_POINT ( 'NONE',  ( 4.337826254667723092, 52.50833866356535395, 24.62149076657007640 ) ) ;
#7437=CARTESIAN_POINT ( 'NONE',  ( 0.6651180000198534392, 9.999999999999987566, 21.00000000000000000 ) ) ;
#7439=CARTESIAN_POINT ( 'NONE',  ( 10.00000000000000355, 20.00000000000000355, -22.91287847477919826 ) ) ;
#7456=CARTESIAN_POINT ( 'NONE',  ( 5.041410851502566182, 11.35764812998954731, -20.38800383682523076 ) ) ;
#7478=CARTESIAN_POINT ( 'NONE',  ( -10.00000000000000178, 20.32878730486446273, 22.91287847477919826 ) ) ;
#7498=CARTESIAN_POINT ( 'NONE',  ( -4.491762996560707322, 47.77920471472745589, -20.51440311031020158 ) ) ;
#7520=CARTESIAN_POINT ( 'NONE',  ( -9.673467176944807733, 17.38163042592174889, -23.05306748635229752 ) ) ;
#7521=CARTESIAN_POINT ( 'NONE',  ( 4.468390986973521883, 11.04793033951060011, -20.52120868300845657 ) ) ;
#7534=CARTESIAN_POINT ( 'NONE',  ( -9.739271384326251280, 22.29254948852628715, -18.60516067502140558 ) ) ;
#7546=VERTEX_POINT ( 'NONE', #7128 ) ;
#7547=CARTESIAN_POINT ( 'NONE',  ( 3.061616997868383043E-15, 139.9999999999999716, 25.00000000000000000 ) ) ;
#7563=CARTESIAN_POINT ( 'NONE',  ( 6.106435932944510370, 12.07435209537243814, 20.09427717736598851 ) ) ;
#7578=CARTESIAN_POINT ( 'NONE',  ( 6.612460753110299017, 12.47060822435505756, 24.11434807139940517 ) ) ;
#7599=CARTESIAN_POINT ( 'NONE',  ( -5.045054645757931944, 28.65860100811472932, -20.39267833245444805 ) ) ;
#7608=CARTESIAN_POINT ( 'NONE',  ( 10.00000000000000355, 20.00000000000000355, -18.46618531261938401 ) ) ;
#7624=CARTESIAN_POINT ( 'NONE',  ( -4.967050660446461485, 49.34001764944455459, -20.40423414033599059 ) ) ;
#7637=CARTESIAN_POINT ( 'NONE',  ( -4.461205683540790723, 28.97367431253432812, -24.60633856694852994 ) ) ;
#7647=CARTESIAN_POINT ( 'NONE',  ( 1.328610784013299906, 10.08300648071286254, -20.96057967355971385 ) ) ;
#7662=CARTESIAN_POINT ( 'NONE',  ( -7.933240127388049068, 26.09654486848563337, -19.44510781892114437 ) ) ;
#7689=CARTESIAN_POINT ( 'NONE',  ( 5.844014480200539374, 11.87882549901748241, 20.17240906330831507 ) ) ;
#7698=CARTESIAN_POINT ( 'NONE',  ( -7.533608174404544222, 26.60766787979761006, -23.84262432367340523 ) ) ;
#7709=CARTESIAN_POINT ( 'NONE',  ( 8.962973916282662046, 15.55345101320112455, -18.99194879768439037 ) ) ;
#7723=CARTESIAN_POINT ( 'NONE',  ( 3.307665144821749337, 53.76359313335627377, -20.73917751733423742 ) ) ;
#7725=ORIENTED_EDGE ( 'NONE', *, *, #10992, .F. ) ;
#7734=CARTESIAN_POINT ( 'NONE',  ( 8.648708627877683242, 25.03051607003104095, -19.13710648617777466 ) ) ;
#7760=DIRECTION ( 'NONE',  ( 0.000000000000000000, -0.000000000000000000, 1.000000000000000000 ) ) ;
#7761=ORIENTED_EDGE ( 'NONE', *, *, #3642, .T. ) ;
#7817=LINE ( 'NONE', #5854, #2973 ) ;
#7826=PLANE ( 'NONE',  #5048 ) ;
#7834=DIRECTION ( 'NONE',  ( -0.000000000000000000, -0.000000000000000000, 1.000000000000000000 ) ) ;
#7843=CARTESIAN_POINT ( 'NONE',  ( 3.761098173404043621, 53.29862245996868353, -24.71568690466639140 ) ) ;
#7885=CARTESIAN_POINT ( 'NONE',  ( -9.659227801817477754, 22.60918507870266581, -23.05884188866823337 ) ) ;
#7890=CARTESIAN_POINT ( 'NONE',  ( 2.213389590484158731, 45.51360200414269741, -24.90224851187377553 ) ) ;
#7907=CYLINDRICAL_SURFACE ( 'NONE', #1536, 10.00000000000000355 ) ;
#7919=CARTESIAN_POINT ( 'NONE',  ( 9.669242541481478881, 22.63421706188354676, 18.64209396758665349 ) ) ;
#7926=CARTESIAN_POINT ( 'NONE',  ( 2.611671490993349831, 29.65850121673988227, -24.86521292532985328 ) ) ;
#7930=EDGE_CURVE ( 'NONE', #7940, #11698, #3880, .T. ) ;
#7937=VERTEX_POINT ( 'NONE', #398 ) ;
#7940=VERTEX_POINT ( 'NONE', #7174 ) ;
#7953=ORIENTED_EDGE ( 'NONE', *, *, #4175, .T. ) ;
#7955=CARTESIAN_POINT ( 'NONE',  ( 1.614286760591197245, 45.25655306502918762, -24.94965407877490549 ) ) ;
#7957=VERTEX_POINT ( 'NONE', #3368 ) ;
#7965=CARTESIAN_POINT ( 'NONE',  ( -8.646677694484681709, 25.03392565432033479, 19.13801979030388267 ) ) ;
#7969=CARTESIAN_POINT ( 'NONE',  ( 4.840263798742708623, 51.29555919482307758, -24.52704763417973410 ) ) ;
#7973=EDGE_CURVE ( 'NONE', #2695, #11970, #9090, .T. ) ;
#7983=CARTESIAN_POINT ( 'NONE',  ( -2.217037138455994150, 45.50647851044359982, -24.90334479454202921 ) ) ;
#7985=CARTESIAN_POINT ( 'NONE',  ( 0.6704130607590332858, 30.00000000000001421, -21.00000000000000355 ) ) ;
#8007=CARTESIAN_POINT ( 'NONE',  ( -2.220795175011430533, 54.49171124227147089, -24.90301599942658228 ) ) ;
#8018=CARTESIAN_POINT ( 'NONE',  ( 0.6521974589784806930, 45.03172573485493047, -24.99359419162020757 ) ) ;
#8020=CARTESIAN_POINT ( 'NONE',  ( 4.840015692395701841, 51.29662771565712376, -20.43473901115169156 ) ) ;
#8031=CARTESIAN_POINT ( 'NONE',  ( -0.3305617426509971923, 30.00000000000001421, 21.00000000000000355 ) ) ;
#8035=CARTESIAN_POINT ( 'NONE',  ( 4.067198847596982247, 52.91284127144104588, -24.66711128229975003 ) ) ;
#8037=DIRECTION ( 'NONE',  ( -0.000000000000000000, -0.000000000000000000, 1.000000000000000000 ) ) ;
#8039=CARTESIAN_POINT ( 'NONE',  ( -9.736206060811452900, 17.69460112315557510, -18.60676615975237880 ) ) ;
#8048=CARTESIAN_POINT ( 'NONE',  ( -4.555463605440090546, 47.93247208080379806, -24.58153461361902359 ) ) ;
#8070=ORIENTED_EDGE ( 'NONE', *, *, #5608, .F. ) ;
#8072=CARTESIAN_POINT ( 'NONE',  ( -4.743369866101525112, 51.61445767325203349, -24.54621253249761637 ) ) ;
#8103=CARTESIAN_POINT ( 'NONE',  ( -8.968054450094975039, 15.52726727364191994, -18.99089028591819428 ) ) ;
#8104=CARTESIAN_POINT ( 'NONE',  ( 4.153883524164314167, 10.89765663934413276, -24.65439000785841372 ) ) ;
#8110=CARTESIAN_POINT ( 'NONE',  ( 4.164372531543180322, 29.09754760689071063, 20.58525091202328738 ) ) ;
#8118=CARTESIAN_POINT ( 'NONE',  ( 5.000000000000000000, 50.33107439471904598, 24.49489742783178770 ) ) ;
#8125=VERTEX_POINT ( 'NONE', #9462 ) ;
#8128=CARTESIAN_POINT ( 'NONE',  ( 6.955575927950914131E-22, 45.00000000000000711, -25.00000000000000000 ) ) ;
#8162=VERTEX_POINT ( 'NONE', #5591 ) ;
#8167=CARTESIAN_POINT ( 'NONE',  ( 6.114177788104627531, 12.06044222946883693, -24.24708634001311580 ) ) ;
#8177=CARTESIAN_POINT ( 'NONE',  ( 4.742699133420079427, 48.38316774318188607, 20.45784509570819765 ) ) ;
#8180=CARTESIAN_POINT ( 'NONE',  ( 4.743169864344128683, 48.38453593858750423, 24.54625634892152775 ) ) ;
#8210=ORIENTED_EDGE ( 'NONE', *, *, #5907, .T. ) ;
#8227=CARTESIAN_POINT ( 'NONE',  ( 5.000000000000000000, 50.33148762970345302, 20.39607805437114507 ) ) ;
#8228=CARTESIAN_POINT ( 'NONE',  ( 9.482520708152488709, 16.75818430496380529, -23.13341755400983502 ) ) ;
#8233=CARTESIAN_POINT ( 'NONE',  ( -5.038456156925416707, 11.33776630238819116, 24.49323865847078707 ) ) ;
#8235=SHAPE_REPRESENTATION ( 'Support Axle', ( #9021 ), #3536 ) ;
#8236=CARTESIAN_POINT ( 'NONE',  ( -3.255256241227468372, 10.53893016368868096, 20.74860095102915736 ) ) ;
#8267=CARTESIAN_POINT ( 'NONE',  ( -4.336726535208759614, 47.49029485220934532, 24.62166619875052831 ) ) ;
#8271=LINE ( 'NONE', #10175, #2524 ) ;
#8288=CARTESIAN_POINT ( 'NONE',  ( -9.868061339005878452, 18.34793401400264301, -22.97011835729309936 ) ) ;
#8289=CARTESIAN_POINT ( 'NONE',  ( 7.946724766127979400, 13.89530605390606688, -23.70643652970303350 ) ) ;
#8295=CARTESIAN_POINT ( 'NONE',  ( -9.983814731900727324, 19.34254964819328038, 22.91996290304706108 ) ) ;
#8299=CARTESIAN_POINT ( 'NONE',  ( 10.00000000000000355, 20.00000000000000355, 22.91287847477919826 ) ) ;
#8305=CARTESIAN_POINT ( 'NONE',  ( 4.338021161404794768, 47.49236434914906368, 24.62144314154611990 ) ) ;
#8306=CARTESIAN_POINT ( 'NONE',  ( 3.419345135684301873, 53.65163791593241172, 24.76532955609361863 ) ) ;
#8333=EDGE_LOOP ( 'NONE', ( #8070, #6318, #11392, #2233, #11138, #9588 ) ) ;
#8348=ORIENTED_EDGE ( 'NONE', *, *, #5812, .F. ) ;
#8357=CARTESIAN_POINT ( 'NONE',  ( -0.3323029841801601880, 10.00000000000000711, 20.99999999999999645 ) ) ;
#8358=CARTESIAN_POINT ( 'NONE',  ( 0.000000000000000000, 0.000000000000000000, 0.000000000000000000 ) ) ;
#8361=CARTESIAN_POINT ( 'NONE',  ( -1.297965663867492347, 54.83959394270241461, 24.96833505342767978 ) ) ;
#8364=CARTESIAN_POINT ( 'NONE',  ( 3.045782272221063902, 53.96862488584907425, 24.81409817615884705 ) ) ;
#8393=CARTESIAN_POINT ( 'NONE',  ( 4.462820119357231441, 11.02737396841608586, 20.52942579431584846 ) ) ;
#8407=CARTESIAN_POINT ( 'NONE',  ( 9.933637772289912959, 18.67556250305220189, 22.94215742280771408 ) ) ;
#8418=CARTESIAN_POINT ( 'NONE',  ( -6.124501814769208075, 12.06839632704649112, 20.09480714311373362 ) ) ;
#8421=CARTESIAN_POINT ( 'NONE',  ( 7.298955741910466699, 26.84326632351102759, 23.91197098918000918 ) ) ;
#8424=CARTESIAN_POINT ( 'NONE',  ( 3.061617023331388775E-15, 45.00000000000000711, 25.00000000000000000 ) ) ;
#8446=CARTESIAN_POINT ( 'NONE',  ( 2.562745747226488176E-15, 30.00000000000001066, 21.00000000000000000 ) ) ;
#8451=AXIS2_PLACEMENT_3D ( 'NONE', #872, #8611, #3660 ) ;
#8453=APPLICATION_CONTEXT ( 'automotive_design' ) ;
#8463=CARTESIAN_POINT ( 'NONE',  ( -5.033342733373901368, 28.66546597776486038, -24.49435860509168350 ) ) ;
#8472=CARTESIAN_POINT ( 'NONE',  ( 3.050582886893512313, 53.97508389715062549, 20.77906331675102081 ) ) ;
#8473=CARTESIAN_POINT ( 'NONE',  ( 5.318519735642854407, 11.52546059409457513, -20.31725095129150560 ) ) ;
#8483=CARTESIAN_POINT ( 'NONE',  ( -4.968274749745848595, 50.65218571871033504, 24.50144017370611493 ) ) ;
#8495=CARTESIAN_POINT ( 'NONE',  ( 1.615386348054266508, 45.25691898032514615, -20.93996090919613096 ) ) ;
#8498=ORIENTED_EDGE ( 'NONE', *, *, #10992, .T. ) ;
#8509=CARTESIAN_POINT ( 'NONE',  ( -4.335701919804127336, 47.48856945494961224, -20.54837457294841130 ) ) ;
#8512=CARTESIAN_POINT ( 'NONE',  ( 1.321940027897182901, 10.06569995984262356, 20.96847759216316476 ) ) ;
#8522=CARTESIAN_POINT ( 'NONE',  ( -3.709758735690515970E-18, 30.00000000000001066, -25.00000000000000000 ) ) ;
#8526=CARTESIAN_POINT ( 'NONE',  ( 9.465993554759519313, 16.75899710733777326, 23.13883973029316010 ) ) ;
#8556=CARTESIAN_POINT ( 'NONE',  ( -3.973477254255321167, 53.05279027209265763, -20.62149924635092546 ) ) ;
#8573=CARTESIAN_POINT ( 'NONE',  ( -3.974164006894358003, 46.94850610908187605, -20.62134886892444641 ) ) ;
#8578=CARTESIAN_POINT ( 'NONE',  ( 5.340684424226280325E-17, 55.00000000000000000, -25.00000000000000000 ) ) ;
#8594=CARTESIAN_POINT ( 'NONE',  ( 7.945130733125017386, 13.89325898989267571, -19.44295271810430847 ) ) ;
#8611=DIRECTION ( 'NONE',  ( 0.000000000000000000, 1.000000000000000000, 0.000000000000000000 ) ) ;
#8615=CARTESIAN_POINT ( 'NONE',  ( -4.493388836263841668, 52.21708239239048055, -20.51403955935326096 ) ) ;
#8629=CYLINDRICAL_SURFACE ( 'NONE', #192, 5.000000000000000000 ) ;
#8650=CARTESIAN_POINT ( 'NONE',  ( 7.927224944456558120, 13.89552811154835510, 23.71088769051724654 ) ) ;
#8654=EDGE_CURVE ( 'NONE', #11587, #8715, #11257, .T. ) ;
#8657=CARTESIAN_POINT ( 'NONE',  ( 6.855064305785296241, 12.71219435950246712, -19.85111039280309342 ) ) ;
#8673=B_SPLINE_CURVE_WITH_KNOTS ( 'NONE', 3,
 ( #7342, #12232, #7220, #10316, #8180, #2458, #8305, #442, #4488, #5453, #4303, #3476, #11091, #6333, #4551, #11344, #2397, #8424 ),
 .UNSPECIFIED., .F., .F.,
 ( 4, 2, 2, 2, 2, 2, 2, 2, 4 ),
 ( 0.000000000000000000, 0.0009797303413002214287, 0.001959460682600442857, 0.002939191023900664286, 0.003918921365200885715, 0.004898651706501107143, 0.005878382047801328572, 0.006858112389101550001, 0.007837842730401771429 ),
 .UNSPECIFIED. ) ;
#8676=EDGE_CURVE ( 'NONE', #332, #12540, #6119, .T. ) ;
#8682=CARTESIAN_POINT ( 'NONE',  ( 9.099857169894804088, 24.15926487358204611, -18.92649755607681783 ) ) ;
#8685=CARTESIAN_POINT ( 'NONE',  ( 0.3338900548043083893, 30.00000000000001066, -25.00000000000000355 ) ) ;
#8710=CARTESIAN_POINT ( 'NONE',  ( -9.355575343945487177, 23.54668771876638189, -23.18385937405269459 ) ) ;
#8714=CARTESIAN_POINT ( 'NONE',  ( 1.314997555680467389, 10.06486170053814533, 24.97384176433527969 ) ) ;
#8715=VERTEX_POINT ( 'NONE', #1864 ) ;
#8741=CARTESIAN_POINT ( 'NONE',  ( 0.3269974554053095006, 45.00000000000000711, -20.99999999999999289 ) ) ;
#8742=CARTESIAN_POINT ( 'NONE',  ( 7.929954359405766873, 26.10079283832167008, -19.44644565266314373 ) ) ;
#8745=CARTESIAN_POINT ( 'NONE',  ( 6.601689117734505174, 27.51820487403981375, -24.11400268645312650 ) ) ;
#8758=EDGE_LOOP ( 'NONE', ( #6824, #9983, #937, #5896, #3972, #11743 ) ) ;
#8769=ORIENTED_EDGE ( 'NONE', *, *, #12103, .T. ) ;
#8789=CARTESIAN_POINT ( 'NONE',  ( 4.339699721346885752, 52.50479725378321660, -24.62114839412567235 ) ) ;
#8798=EDGE_CURVE ( 'NONE', #7546, #8162, #4741, .T. ) ;
#8803=CARTESIAN_POINT ( 'NONE',  ( -4.744081181139592651, 48.38712208294071360, -24.54608042500704457 ) ) ;
#8806=ORIENTED_EDGE ( 'NONE', *, *, #1174, .F. ) ;
#8807=CARTESIAN_POINT ( 'NONE',  ( 4.462630933173456604, 28.97330998342967234, -24.60619142875309251 ) ) ;
#8822=VERTEX_POINT ( 'NONE', #10677 ) ;
#8823=CARTESIAN_POINT ( 'NONE',  ( -4.339203347172030156, 52.50587310092982563, -24.62124401584528499 ) ) ;
#8848=ORIENTED_EDGE ( 'NONE', *, *, #11416, .T. ) ;
#8854=DIRECTION ( 'NONE',  ( 1.000000000000000000, 0.000000000000000000, 0.000000000000000000 ) ) ;
#8861=ADVANCED_FACE ( 'NONE', ( #987 ), #3959, .F. ) ;
#8867=CARTESIAN_POINT ( 'NONE',  ( -1.301064515050044168, 45.16113941612564275, -24.96819193944210724 ) ) ;
#8891=CARTESIAN_POINT ( 'NONE',  ( -1.615502922434717492, 54.74315837822297937, -24.94959493428010688 ) ) ;
#8898=CARTESIAN_POINT ( 'NONE',  ( -9.466558637120989772, 23.23925856829589520, -23.13860710034107626 ) ) ;
#8913=CARTESIAN_POINT ( 'NONE',  ( -9.917191296150036806, 21.32702561569567834, 18.51082767248323080 ) ) ;
#8917=CARTESIAN_POINT ( 'NONE',  ( 4.967652032308136789, 50.65502714036492904, -24.50156428836015721 ) ) ;
#8934=CARTESIAN_POINT ( 'NONE',  ( -4.245899883333350111, 47.35448134532762055, -24.63697916171703994 ) ) ;
#8936=EDGE_CURVE ( 'NONE', #11306, #1221, #5805, .T. ) ;
#8939=CARTESIAN_POINT ( 'NONE',  ( 3.763916608749744874, 46.69265501667148044, 20.66125156366808113 ) ) ;
#8967=CARTESIAN_POINT ( 'NONE',  ( 2.286402882168606432, 10.25929110584701931, 24.89734643733720176 ) ) ;
#8968=ORIENTED_EDGE ( 'NONE', *, *, #6919, .F. ) ;
#8975=DIRECTION ( 'NONE',  ( -0.000000000000000000, -1.000000000000000000, -0.000000000000000000 ) ) ;
#8980=CARTESIAN_POINT ( 'NONE',  ( -0.6610962637957030763, 29.98365020075052811, 20.99219928172843197 ) ) ;
#8988=CARTESIAN_POINT ( 'NONE',  ( -2.623156034030268202, 10.34458332881492559, -20.83793945939456549 ) ) ;
#8997=CARTESIAN_POINT ( 'NONE',  ( 5.315759107678847073, 28.47626550783180477, 20.31797234239212102 ) ) ;
#8999=CARTESIAN_POINT ( 'NONE',  ( 6.615359460987012774, 27.52709606376180318, -19.93674538982958211 ) ) ;
#9004=CARTESIAN_POINT ( 'NONE',  ( 5.000000000000000000, 50.00000000000000000, 20.39607805437114152 ) ) ;
#9021=AXIS2_PLACEMENT_3D ( 'NONE', #11433, #2744, #207 ) ;
#9023=ORIENTED_EDGE ( 'NONE', *, *, #8654, .F. ) ;
#9041=PRODUCT ( 'Support Axle', 'Support Axle', '', ( #1147 ) ) ;
#9047=CARTESIAN_POINT ( 'NONE',  ( 5.000000000000000000, 50.00000000000000000, 20.39607805437114152 ) ) ;
#9052=ORIENTED_EDGE ( 'NONE', *, *, #6526, .T. ) ;
#9058=CARTESIAN_POINT ( 'NONE',  ( 9.673501139021151829, 17.38172013086462542, -23.05305332146628317 ) ) ;
#9064=CARTESIAN_POINT ( 'NONE',  ( -1.299587538611466586, 54.83916993575238052, 20.96219696135102595 ) ) ;
#9067=LINE ( 'NONE', #10829, #5790 ) ;
#9071=EDGE_CURVE ( 'NONE', #12540, #8162, #597, .T. ) ;
#9085=ORIENTED_EDGE ( 'NONE', *, *, #7341, .F. ) ;
#9090=LINE ( 'NONE', #6292, #12417 ) ;
#9118=VERTEX_POINT ( 'NONE', #4646 ) ;
#9120=CARTESIAN_POINT ( 'NONE',  ( -8.961327849752377617, 24.44988401922752530, 23.33927995079777062 ) ) ;
#9123=LINE ( 'NONE', #6263, #4629 ) ;
#9139=CARTESIAN_POINT ( 'NONE',  ( 3.061617023331388775E-15, 45.00000000000000711, 25.00000000000000000 ) ) ;
#9162=EDGE_LOOP ( 'NONE', ( #12109, #7327, #3018, #12089, #1178, #5940, #10720, #3184, #11185, #5924, #467, #10344, #11570, #2061, #4533, #11658 ) ) ;
#9164=VERTEX_POINT ( 'NONE', #12450 ) ;
#9177=ORIENTED_EDGE ( 'NONE', *, *, #8798, .T. ) ;
#9182=CARTESIAN_POINT ( 'NONE',  ( 8.963427797786382101, 15.55435157282535741, -23.33847234685102379 ) ) ;
#9191=CARTESIAN_POINT ( 'NONE',  ( 1.313665803496629980, 29.93556061881280428, 24.97400592093060112 ) ) ;
#9193=CARTESIAN_POINT ( 'NONE',  ( 4.967314895201458746, 49.34232189057839690, 20.40416878132349510 ) ) ;
#9214=DIRECTION ( 'NONE',  ( -0.000000000000000000, -1.000000000000000000, -0.000000000000000000 ) ) ;
#9223=CARTESIAN_POINT ( 'NONE',  ( -0.3269774092232215490, 45.00000000000000000, 25.00000000000000711 ) ) ;
#9245=CARTESIAN_POINT ( 'NONE',  ( -7.929079634139357680, 13.89786668772332767, -23.71027527960010417 ) ) ;
#9246=CARTESIAN_POINT ( 'NONE',  ( -3.243418093453738216, 29.48203249043655561, 24.79625640031606082 ) ) ;
#9251=CARTESIAN_POINT ( 'NONE',  ( -8.967015720386880773, 15.56160195868188545, 23.33709189419391805 ) ) ;
#9258=EDGE_LOOP ( 'NONE', ( #10174, #9737, #980, #9177, #1299, #3776 ) ) ;
#9272=VERTEX_POINT ( 'NONE', #10786 ) ;
#9273=CARTESIAN_POINT ( 'NONE',  ( 2.562745747226488176E-15, 30.00000000000001066, 21.00000000000000000 ) ) ;
#9305=ORIENTED_EDGE ( 'NONE', *, *, #747, .F. ) ;
#9307=CARTESIAN_POINT ( 'NONE',  ( -8.483825669166648709, 25.30371668182424827, 23.51725424962153355 ) ) ;
#9309=DIRECTION ( 'NONE',  ( -0.000000000000000000, -1.000000000000000000, -0.000000000000000000 ) ) ;
#9310=CLOSED_SHELL ( 'NONE', ( #4217, #6712, #8861, #1412, #11705, #9857, #5023, #10137, #1784, #5587, #11168, #797, #3627, #6042 ) ) ;
#9314=DIRECTION ( 'NONE',  ( -0.000000000000000000, -1.000000000000000000, -0.000000000000000000 ) ) ;
#9318=CARTESIAN_POINT ( 'NONE',  ( 10.00000000000000888, 20.33378987232122981, 22.91287847477920536 ) ) ;
#9320=CARTESIAN_POINT ( 'NONE',  ( -4.556215257066872582, 52.06578128350423640, 24.58139409886873139 ) ) ;
#9324=CARTESIAN_POINT ( 'NONE',  ( 2.912936886510098855, 54.06713064528141643, 24.83009325023465763 ) ) ;
#9344=CARTESIAN_POINT ( 'NONE',  ( -3.256860162955865334, 29.47720352819935030, 20.75492283549158401 ) ) ;
#9351=CARTESIAN_POINT ( 'NONE',  ( 10.00000000000000178, 19.32777951161647323, 18.46618531261938756 ) ) ;
#9354=AXIS2_PLACEMENT_3D ( 'NONE', #5353, #6239, #10231 ) ;
#9365=CARTESIAN_POINT ( 'NONE',  ( 10.00000000000000533, 19.33140358361892552, 22.91287847477920891 ) ) ;
#9366=ORIENTED_EDGE ( 'NONE', *, *, #8676, .T. ) ;
#9369=EDGE_CURVE ( 'NONE', #8125, #2736, #7817, .T. ) ;
#9370=CARTESIAN_POINT ( 'NONE',  ( -8.122732253212674891, 14.15824396964088372, -23.64440389997412950 ) ) ;
#9371=CARTESIAN_POINT ( 'NONE',  ( 6.613906629224937106, 12.49257982187926785, -19.93301561218848761 ) ) ;
#9373=CYLINDRICAL_SURFACE ( 'NONE', #1106, 10.00000000000000355 ) ;
#9375=CARTESIAN_POINT ( 'NONE',  ( -9.737903098387532097, 17.70124625263684592, 18.60587983635906539 ) ) ;
#9379=CARTESIAN_POINT ( 'NONE',  ( -3.049660161009143611, 53.97562969122508747, 24.81478968795947537 ) ) ;
#9391=CYLINDRICAL_SURFACE ( 'NONE', #2109, 21.00000000000000000 ) ;
#9393=DIRECTION ( 'NONE',  ( -0.000000000000000000, -0.000000000000000000, 1.000000000000000000 ) ) ;
#9394=CARTESIAN_POINT ( 'NONE',  ( 0.000000000000000000, 50.00000000000000000, -28.00000000000000711 ) ) ;
#9402=EDGE_CURVE ( 'NONE', #1221, #5152, #8673, .T. ) ;
#9403=CARTESIAN_POINT ( 'NONE',  ( -1.654777828561690312, 29.86772917176804398, 20.93725631092291906 ) ) ;
#9408=CARTESIAN_POINT ( 'NONE',  ( -3.051146662956820688, 46.02554824080852569, -20.77895220992095560 ) ) ;
#9411=CARTESIAN_POINT ( 'NONE',  ( 2.619390655685069014, 10.34347335722847916, 20.83845118924497086 ) ) ;
#9422=CARTESIAN_POINT ( 'NONE',  ( -2.610103423518925769, 29.65902056345734650, -24.86541183722168213 ) ) ;
#9430=CARTESIAN_POINT ( 'NONE',  ( 4.337336347961448624, 52.50902530749537078, 20.54804625155474440 ) ) ;
#9431=CARTESIAN_POINT ( 'NONE',  ( 10.00000000000000355, 20.00000000000000355, -18.46618531261938401 ) ) ;
#9439=CARTESIAN_POINT ( 'NONE',  ( 7.519126441075570710, 26.60062706338189642, 23.84344315696457173 ) ) ;
#9441=ORIENTED_EDGE ( 'NONE', *, *, #2201, .T. ) ;
#9444=B_SPLINE_CURVE_WITH_KNOTS ( 'NONE', 3,
 ( #808, #9569, #5762, #4742, #9631, #746, #4681, #941, #7599, #5823, #11660, #12479, #4870, #2773, #3782, #7662, #6702, #10569, #9607, #6576, #6831, #3659, #7534, #11402, #2712, #10441 ),
 .UNSPECIFIED., .F., .F.,
 ( 4, 2, 2, 2, 2, 2, 2, 2, 2, 2, 2, 2, 4 ),
 ( 3.701750345114177145E-18, 0.001985659510702812366, 0.002978489266054215080, 0.003971319021405616927, 0.005956978532108423222, 0.006949808287459825068, 0.007942638042811226914, 0.008935467798162625291, 0.009928297553514025403, 0.01191395706421683257, 0.01290678681956823615, 0.01389961657491964146, 0.01588527608562245730 ),
 .UNSPECIFIED. ) ;
#9445=ADVANCED_BREP_SHAPE_REPRESENTATION ( '', ( #2150, #9021 ), #3536 ) ;
#9453=DIRECTION ( 'NONE',  ( -0.000000000000000000, -0.000000000000000000, 1.000000000000000000 ) ) ;
#9462=CARTESIAN_POINT ( 'NONE',  ( 0.000000000000000000, 139.9999999999999716, -21.00000000000000000 ) ) ;
#9474=ORIENTED_EDGE ( 'NONE', *, *, #10533, .T. ) ;
#9483=CARTESIAN_POINT ( 'NONE',  ( -3.242423582264189807, 29.46551675503955536, -24.79088612835948879 ) ) ;
#9488=CARTESIAN_POINT ( 'NONE',  ( 9.353363810095283171, 16.44731154698707698, 23.18475774758237407 ) ) ;
#9520=LINE ( 'NONE', #7547, #6909 ) ;
#9528=FACE_OUTER_BOUND ( 'NONE', #4992, .T. ) ;
#9530=ORIENTED_EDGE ( 'NONE', *, *, #4175, .F. ) ;
#9535=CARTESIAN_POINT ( 'NONE',  ( 5.033147323133203344, 11.33447346640459230, 20.39563185274203150 ) ) ;
#9538=DIRECTION ( 'NONE',  ( 0.000000000000000000, 0.000000000000000000, 1.000000000000000000 ) ) ;
#9551=CARTESIAN_POINT ( 'NONE',  ( 10.00000000000000355, 20.00000000000000355, 22.91287847477919826 ) ) ;
#9555=CARTESIAN_POINT ( 'NONE',  ( 7.538096365933896870, 13.39748730115788966, -19.60640367412442231 ) ) ;
#9558=CARTESIAN_POINT ( 'NONE',  ( -4.743623831329197849, 48.38606213893405794, 20.45762700453146721 ) ) ;
#9565=CARTESIAN_POINT ( 'NONE',  ( 4.743041305584357659, 51.61559430690765282, -20.45776197285908538 ) ) ;
#9569=CARTESIAN_POINT ( 'NONE',  ( -0.6720848162426399375, 30.00000000000001776, -21.00000000000000711 ) ) ;
#9570=FACE_OUTER_BOUND ( 'NONE', #9911, .T. ) ;
#9588=ORIENTED_EDGE ( 'NONE', *, *, #3384, .F. ) ;
#9591=ORIENTED_EDGE ( 'NONE', *, *, #6919, .T. ) ;
#9607=CARTESIAN_POINT ( 'NONE',  ( -8.975987864778222303, 24.45580491392657052, -18.98708776393284836 ) ) ;
#9609=CARTESIAN_POINT ( 'NONE',  ( 9.739739614376460963, 17.70973893131317922, 23.02482158226496622 ) ) ;
#9621=CARTESIAN_POINT ( 'NONE',  ( -3.974643129415062148, 46.94910658706874784, 20.62125717344303411 ) ) ;
#9631=CARTESIAN_POINT ( 'NONE',  ( -2.621352440196214495, 29.65601317703552198, -20.83821235188215226 ) ) ;
#9632=EDGE_CURVE ( 'NONE', #11970, #1856, #9444, .T. ) ;
#9639=CARTESIAN_POINT ( 'NONE',  ( 9.478213219505041920, 23.25438371585110886, -18.74145979309692578 ) ) ;
#9643=CARTESIAN_POINT ( 'NONE',  ( 7.532348232781783892, 26.60942912475959332, -23.84307605514715434 ) ) ;
#9660=EDGE_LOOP ( 'NONE', ( #9591, #4836 ) ) ;
#9673=CARTESIAN_POINT ( 'NONE',  ( 2.502435999373153308, 45.66817884423451801, -24.87486459250430926 ) ) ;
#9700=LINE ( 'NONE', #5769, #7157 ) ;
#9701=CARTESIAN_POINT ( 'NONE',  ( 8.122033900404826312, 25.84264039288823511, -19.36674556122184399 ) ) ;
#9705=CARTESIAN_POINT ( 'NONE',  ( 9.466290622766221574, 23.23991477998078636, -23.13871526284164304 ) ) ;
#9714=DIRECTION ( 'NONE',  ( 1.000000000000000000, 0.000000000000000000, 0.000000000000000000 ) ) ;
#9723=DIRECTION ( 'NONE',  ( -0.000000000000000000, -1.000000000000000000, -0.000000000000000000 ) ) ;
#9737=ORIENTED_EDGE ( 'NONE', *, *, #2977, .T. ) ;
#9762=CARTESIAN_POINT ( 'NONE',  ( 5.038105599187825412, 28.64433225779773551, 20.38884022818624331 ) ) ;
#9763=CARTESIAN_POINT ( 'NONE',  ( 4.336879845426758529, 47.49058353134505950, -20.54812575080782011 ) ) ;
#9766=ORIENTED_EDGE ( 'NONE', *, *, #11531, .T. ) ;
#9783=SHAPE_REPRESENTATION_RELATIONSHIP ( 'NONE' , 'NONE' ,  #8235, #9445 ) ;
#9795=B_SPLINE_CURVE_WITH_KNOTS ( 'NONE', 3,
 ( #11490, #9351, #772, #1779, #2677, #6663, #12446, #5727, #12506, #2799, #10345, #1843, #4641, #3809, #6540, #7563, #7689, #9535, #8393, #653, #12262, #9411, #3562, #8512, #7437, #1722 ),
 .UNSPECIFIED., .F., .F.,
 ( 4, 2, 2, 2, 2, 2, 2, 2, 2, 2, 2, 2, 4 ),
 ( 0.000000000000000000, 0.001985162064921483505, 0.002977743097382220486, 0.003970324129842958336, 0.005955486194764421023, 0.006948067227225150633, 0.007940648259685878507, 0.008933229292146606382, 0.009925810324607334256, 0.01191097238952878480, 0.01290355342198951268, 0.01389613445445023708, 0.01588129651937168763 ),
 .UNSPECIFIED. ) ;
#9798=CARTESIAN_POINT ( 'NONE',  ( 4.450527323037263727, 11.02130320606087821, 24.60818795580814822 ) ) ;
#9826=CARTESIAN_POINT ( 'NONE',  ( -4.838879514055022923, 48.69911239754581089, -24.52732196506755713 ) ) ;
#9827=CARTESIAN_POINT ( 'NONE',  ( 4.935074631655826494, 49.18045323697044324, -20.41191120140011606 ) ) ;
#9828=CARTESIAN_POINT ( 'NONE',  ( 4.464751531075205726, 28.95392510639267414, -20.52201552506329918 ) ) ;
#9849=CARTESIAN_POINT ( 'NONE',  ( -3.307156092220256749, 53.76411647547837447, -24.78137765757908895 ) ) ;
#9857=ADVANCED_FACE ( 'NONE', ( #11847 ), #1133, .T. ) ;
#9876=CARTESIAN_POINT ( 'NONE',  ( 0.6578411763953998515, 54.96743791211429908, -24.99342793576595767 ) ) ;
#9883=CARTESIAN_POINT ( 'NONE',  ( -9.916489090768509485, 18.66787674250353390, -18.51120417158414000 ) ) ;
#9889=CARTESIAN_POINT ( 'NONE',  ( 0.3302971441079701753, 30.00000000000001776, 21.00000000000000711 ) ) ;
#9890=CARTESIAN_POINT ( 'NONE',  ( -4.493221811708316693, 52.21748163326066106, 20.51407716484954236 ) ) ;
#9894=ORIENTED_EDGE ( 'NONE', *, *, #2271, .F. ) ;
#9896=CARTESIAN_POINT ( 'NONE',  ( 8.484924050289805564, 25.30202893790023921, -23.51686326738786192 ) ) ;
#9911=EDGE_LOOP ( 'NONE', ( #11100, #5528 ) ) ;
#9930=CARTESIAN_POINT ( 'NONE',  ( 5.000000000000000000, 50.00000000000000000, -28.00000000000000711 ) ) ;
#9945=CARTESIAN_POINT ( 'NONE',  ( -7.924078669757784965, 13.89146999950097161, -19.44885958033332329 ) ) ;
#9953=CARTESIAN_POINT ( 'NONE',  ( 8.481018271693534061, 25.30809127690124782, 19.21224764554878917 ) ) ;
#9958=CARTESIAN_POINT ( 'NONE',  ( 1.766134315194576754, 45.31947902013321539, 20.92614565884721145 ) ) ;
#9983=ORIENTED_EDGE ( 'NONE', *, *, #11531, .F. ) ;
#9987=CARTESIAN_POINT ( 'NONE',  ( 4.967692037346607137, 50.65500470054040250, -20.40407670487946135 ) ) ;
#10007=CARTESIAN_POINT ( 'NONE',  ( -0.6619244392933834042, 10.00000000000000178, -21.00000000000000711 ) ) ;
#10016=CARTESIAN_POINT ( 'NONE',  ( 6.955575927950914131E-22, 45.00000000000000711, -25.00000000000000000 ) ) ;
#10017=CARTESIAN_POINT ( 'NONE',  ( 2.559760333650129958E-15, 55.00000000000000000, 21.00000000000000000 ) ) ;
#10024=EDGE_CURVE ( 'NONE', #9272, #1221, #2318, .T. ) ;
#10026=CARTESIAN_POINT ( 'NONE',  ( 4.967437465254620932, 50.65784153438875848, 24.50160996501502098 ) ) ;
#10070=CARTESIAN_POINT ( 'NONE',  ( -9.655198859856366056, 17.37602299191694044, -18.64909941108382796 ) ) ;
#10076=CARTESIAN_POINT ( 'NONE',  ( -0.6688742877673069520, 10.01682275176732162, 20.99197381862867928 ) ) ;
#10079=CARTESIAN_POINT ( 'NONE',  ( 6.119244668491610639, 27.93539859446131501, -20.09633498124250295 ) ) ;
#10114=CARTESIAN_POINT ( 'NONE',  ( 10.00000000000000355, 20.00000000000000355, 22.91287847477919826 ) ) ;
#10131=CARTESIAN_POINT ( 'NONE',  ( 0.000000000000000000, 139.9999999999999716, 0.000000000000000000 ) ) ;
#10134=CARTESIAN_POINT ( 'NONE',  ( -9.866849862893351641, 18.34052833014279216, -18.53781888910907938 ) ) ;
#10135=CARTESIAN_POINT ( 'NONE',  ( 3.061617454482527662E-15, 30.00000000000001066, 25.00000000000000000 ) ) ;
#10137=ADVANCED_FACE ( 'NONE', ( #9570, #5704 ), #2839, .F. ) ;
#10139=CARTESIAN_POINT ( 'NONE',  ( -2.306453115620162198, 10.26403383852864870, 20.87548082228511603 ) ) ;
#10141=CARTESIAN_POINT ( 'NONE',  ( 9.353276081244219498, 23.55311451265283296, 23.18479875781715194 ) ) ;
#10174=ORIENTED_EDGE ( 'NONE', *, *, #100, .F. ) ;
#10175=CARTESIAN_POINT ( 'NONE',  ( 0.000000000000000000, 139.9999999999999716, -21.00000000000000000 ) ) ;
#10190=CARTESIAN_POINT ( 'NONE',  ( 3.972187451669499936, 53.05441016201150717, 20.62174624516992694 ) ) ;
#10191=CARTESIAN_POINT ( 'NONE',  ( -1.322864546895947679, 29.91770977471893289, 24.96717945133217498 ) ) ;
#10192=CARTESIAN_POINT ( 'NONE',  ( 2.571758278209441661E-15, 139.9999999999999716, 21.00000000000000000 ) ) ;
#10194=CARTESIAN_POINT ( 'NONE',  ( -10.00000000000001066, 19.67111324348436696, 22.91287847477920536 ) ) ;
#10202=CARTESIAN_POINT ( 'NONE',  ( 2.504881716134078395, 54.33965200799452333, 24.87570091612971979 ) ) ;
#10223=CARTESIAN_POINT ( 'NONE',  ( -6.116604691219384549, 27.93765947712327247, 20.09721008222173211 ) ) ;
#10231=DIRECTION ( 'NONE',  ( 1.000000000000000000, 0.000000000000000000, 0.000000000000000000 ) ) ;
#10232=ORIENTED_EDGE ( 'NONE', *, *, #12017, .F. ) ;
#10248=CARTESIAN_POINT ( 'NONE',  ( 4.741197079555949934, 51.62084573238831098, 20.45818942849235000 ) ) ;
#10252=CARTESIAN_POINT ( 'NONE',  ( -1.332521848768800865, 10.08356887257211199, 20.96031352669567838 ) ) ;
#10256=CARTESIAN_POINT ( 'NONE',  ( -2.508190414677843982, 54.33763061856527088, 24.87535316732256163 ) ) ;
#10299=( NAMED_UNIT ( * ) PLANE_ANGLE_UNIT ( ) SI_UNIT ( $, .RADIAN. ) );
#10305=CARTESIAN_POINT ( 'NONE',  ( 5.307486386703490489, 11.51851869311760090, -24.43167369944409018 ) ) ;
#10310=FACE_OUTER_BOUND ( 'NONE', #2180, .T. ) ;
#10312=CARTESIAN_POINT ( 'NONE',  ( 9.465308527890080370, 23.24274166418333110, 23.13911695433847981 ) ) ;
#10316=CARTESIAN_POINT ( 'NONE',  ( 4.839779845606726916, 48.70264860999793655, 24.52714343409649089 ) ) ;
#10323=CARTESIAN_POINT ( 'NONE',  ( -9.983825383151277322, 20.65789756057008120, 22.91995855732452370 ) ) ;
#10327=EDGE_LOOP ( 'NONE', ( #7761, #7215, #544, #2976, #3278, #360, #11718, #7291, #3330, #11761, #239, #426, #6406, #4028, #6600, #11485 ) ) ;
#10338=VECTOR ( 'NONE', #9393, 1000.000000000000000 ) ;
#10344=ORIENTED_EDGE ( 'NONE', *, *, #3730, .F. ) ;
#10345=CARTESIAN_POINT ( 'NONE',  ( 7.924332520748174957, 13.89188147265340945, 19.44874353718065763 ) ) ;
#10368=EDGE_CURVE ( 'NONE', #7937, #3410, #355, .T. ) ;
#10370=CARTESIAN_POINT ( 'NONE',  ( 2.571758291765529985E-15, 45.00000000000000711, 21.00000000000000000 ) ) ;
#10375=B_SPLINE_CURVE_WITH_KNOTS ( 'NONE', 3,
 ( #9004, #2145, #9193, #5198, #8177, #11088, #6963, #314, #8939, #2217, #252, #2338, #11856, #9958, #377, #5322, #3228, #3289, #6020, #10970 ),
 .UNSPECIFIED., .F., .F.,
 ( 4, 2, 2, 2, 2, 2, 2, 2, 2, 4 ),
 ( 0.000000000000000000, 0.0009807944672943543635, 0.001961588934588708727, 0.002942383401883063524, 0.003923177869177417454, 0.004903972336471771817, 0.005884766803766127048, 0.006375164037413299893, 0.006865561271060473605, 0.007846355738354819295 ),
 .UNSPECIFIED. ) ;
#10402=CARTESIAN_POINT ( 'NONE',  ( -2.631691148149290171, 29.67035037513104712, 20.84471558130442759 ) ) ;
#10406=CARTESIAN_POINT ( 'NONE',  ( -0.6587939304379992755, 45.03274104319341120, -20.99213535553697341 ) ) ;
#10410=ORIENTED_EDGE ( 'NONE', *, *, #10533, .F. ) ;
#10419=CARTESIAN_POINT ( 'NONE',  ( -10.00000000000000355, 20.00000000000000355, -28.00000000000000711 ) ) ;
#10426=CARTESIAN_POINT ( 'NONE',  ( -5.300214471940789096, 11.51392236371535382, -24.43326627631521220 ) ) ;
#10432=CARTESIAN_POINT ( 'NONE',  ( -1.302025784688028764, 45.16141512708880867, 20.96206104378117985 ) ) ;
#10438=CARTESIAN_POINT ( 'NONE',  ( -5.000000000000000000, 50.32679387323496911, 24.49489742783177704 ) ) ;
#10441=CARTESIAN_POINT ( 'NONE',  ( -10.00000000000000355, 20.00000000000000355, -18.46618531261938401 ) ) ;
#10447=CARTESIAN_POINT ( 'NONE',  ( -5.000000000000000000, 50.00000000000000000, -20.39607805437114152 ) ) ;
#10465=CARTESIAN_POINT ( 'NONE',  ( -1.302315535602271757, 45.16144182297183107, -20.96205453846774347 ) ) ;
#10467=VERTEX_POINT ( 'NONE', #1788 ) ;
#10495=CARTESIAN_POINT ( 'NONE',  ( -3.768782163415854036, 46.69792565062278555, 20.66038494228472899 ) ) ;
#10506=B_SPLINE_CURVE_WITH_KNOTS ( 'NONE', 3,
 ( #3286, #9889, #10698, #6141, #2011, #1259, #6015, #8110, #3030, #9762, #8997, #4238, #6083, #10760, #10966, #9953, #310, #1202, #6895, #1138, #7919, #2140, #5891, #2211 ),
 .UNSPECIFIED., .F., .F.,
 ( 4, 2, 2, 2, 2, 2, 2, 2, 2, 2, 2, 4 ),
 ( 0.04760885841731214013, 0.04859922075612807535, 0.04958958309494400363, 0.05157030777257586712, 0.05256067011139180234, 0.05355103245020773062, 0.05553175712783959411, 0.05751248180547145761, 0.05850284414428739282, 0.05949320648310332110, 0.06147393116073518460, 0.06345465583836705503 ),
 .UNSPECIFIED. ) ;
#10512=LINE ( 'NONE', #878, #3313 ) ;
#10516=DIRECTION ( 'NONE',  ( -0.000000000000000000, -0.000000000000000000, 1.000000000000000000 ) ) ;
#10533=EDGE_CURVE ( 'NONE', #332, #4818, #10664, .T. ) ;
#10544=CARTESIAN_POINT ( 'NONE',  ( -6.108719317430274742, 27.92396576624410187, -24.24357326025485193 ) ) ;
#10546=ORIENTED_EDGE ( 'NONE', *, *, #6826, .T. ) ;
#10566=CARTESIAN_POINT ( 'NONE',  ( 5.000000000000000000, 50.32977410740986812, -20.39607805437114152 ) ) ;
#10569=CARTESIAN_POINT ( 'NONE',  ( -8.670263310646999955, 25.02480281026656073, -19.13064292386552268 ) ) ;
#10576=CARTESIAN_POINT ( 'NONE',  ( 3.303977982198811780, 46.23303585118835457, -20.73977949246337005 ) ) ;
#10580=B_SPLINE_CURVE_WITH_KNOTS ( 'NONE', 3,
 ( #4098, #6010, #4166, #9883, #10134, #8039, #10070, #2204, #12032, #8103, #3337, #3150, #9945, #7201, #1380, #427, #1319, #11910, #11077, #2385, #1254, #1444, #2268, #8988, #5125, #6136, #10007, #5189 ),
 .UNSPECIFIED., .F., .F.,
 ( 4, 2, 2, 2, 2, 2, 2, 2, 2, 2, 2, 2, 2, 4 ),
 ( 0.01588527608562245730, 0.01687704675167533280, 0.01786881741772820831, 0.01886058808378108381, 0.01985235874983395932, 0.02183590008193970339, 0.02282767074799257542, 0.02381944141404544746, 0.02580298274615118459, 0.02679475341220405663, 0.02778652407825692866, 0.02877829474430979723, 0.02977006541036266579, 0.03175360674246840986 ),
 .UNSPECIFIED. ) ;
#10589=CARTESIAN_POINT ( 'NONE',  ( 3.024050948510435495E-21, 45.00000000000000711, -21.00000000000000000 ) ) ;
#10611=CARTESIAN_POINT ( 'NONE',  ( 3.258993009127279628, 10.52298990541062551, -20.75479906574401667 ) ) ;
#10636=CARTESIAN_POINT ( 'NONE',  ( -4.680564368149037868, 51.76601715386365044, -20.47184426876964025 ) ) ;
#10638=CARTESIAN_POINT ( 'NONE',  ( 8.481410126304654185, 25.30750070271793817, -19.21207824733827252 ) ) ;
#10642=CARTESIAN_POINT ( 'NONE',  ( 5.839560020365381021, 28.12428960229776465, -24.30998564924267313 ) ) ;
#10662=CARTESIAN_POINT ( 'NONE',  ( -5.000000000000000000, 50.00000000000000000, -28.00000000000000711 ) ) ;
#10664=LINE ( 'NONE', #12220, #11281 ) ;
#10677=CARTESIAN_POINT ( 'NONE',  ( 2.571758278209441661E-15, 139.9999999999999716, 21.00000000000000000 ) ) ;
#10698=CARTESIAN_POINT ( 'NONE',  ( 0.6606214661398540633, 29.98367637546362019, 20.99221177463937238 ) ) ;
#10716=ORIENTED_EDGE ( 'NONE', *, *, #3245, .T. ) ;
#10720=ORIENTED_EDGE ( 'NONE', *, *, #958, .F. ) ;
#10722=CARTESIAN_POINT ( 'NONE',  ( -4.839726511208201742, 51.29827509403275343, -24.52715513826036897 ) ) ;
#10760=CARTESIAN_POINT ( 'NONE',  ( 7.535696908431325447, 26.60561170258834807, 19.60740232376276637 ) ) ;
#10761=CARTESIAN_POINT ( 'NONE',  ( 5.000000000000000888, 50.00000000000000000, -20.39607805437114152 ) ) ;
#10762=CARTESIAN_POINT ( 'NONE',  ( 5.039783919969697656, 28.64334189333860081, -20.38842086786498342 ) ) ;
#10781=DIRECTION ( 'NONE',  ( 0.000000000000000000, 1.000000000000000000, 0.000000000000000000 ) ) ;
#10786=CARTESIAN_POINT ( 'NONE',  ( 3.061565168526138680E-15, 55.00000000000000000, 25.00000000000000000 ) ) ;
#10792=CARTESIAN_POINT ( 'NONE',  ( -9.740943735563897476, 22.28537929251632477, -23.02431258361445288 ) ) ;
#10794=ORIENTED_EDGE ( 'NONE', *, *, #5812, .T. ) ;
#10798=CARTESIAN_POINT ( 'NONE',  ( 5.000000000000000000, 50.00000000000000000, -24.49489742783178414 ) ) ;
#10807=DIRECTION ( 'NONE',  ( 1.000000000000000000, 0.000000000000000000, 0.000000000000000000 ) ) ;
#10811=CARTESIAN_POINT ( 'NONE',  ( 3.055841136373902422, 53.97118948954670969, -24.81406232681816348 ) ) ;
#10828=CARTESIAN_POINT ( 'NONE',  ( 4.839186675186220477, 48.70048224716990148, -20.43493563430346072 ) ) ;
#10829=CARTESIAN_POINT ( 'NONE',  ( 2.571758278209441661E-15, 139.9999999999999716, 21.00000000000000000 ) ) ;
#10834=CARTESIAN_POINT ( 'NONE',  ( 3.549343885166972523, 29.35473140773891032, -24.74867856782190856 ) ) ;
#10853=EDGE_LOOP ( 'NONE', ( #8769, #8848, #349, #11060, #9530, #1130 ) ) ;
#10863=CARTESIAN_POINT ( 'NONE',  ( -8.673894831530475358, 25.01911591053615425, -23.45021177788830968 ) ) ;
#10874=EDGE_CURVE ( 'NONE', #9164, #11587, #3262, .T. ) ;
#10893=DIRECTION ( 'NONE',  ( -0.000000000000000000, -1.000000000000000000, -0.000000000000000000 ) ) ;
#10935=VERTEX_POINT ( 'NONE', #616 ) ;
#10945=B_SPLINE_CURVE_WITH_KNOTS ( 'NONE', 3,
 ( #6084, #11917, #3224, #2972, #5892, #9890, #5196, #4042, #3160, #7025, #7086, #10967, #2212, #2141, #9064, #3091, #3918, #2275, #6142, #10017 ),
 .UNSPECIFIED., .F., .F.,
 ( 4, 2, 2, 2, 2, 2, 2, 2, 2, 4 ),
 ( 0.01568868358392457724, 0.01666917987226885015, 0.01764967616061312305, 0.01863017244895739596, 0.01961066873730166887, 0.02059116502564593831, 0.02157166131399021469, 0.02255215760233448760, 0.02304240574650662232, 0.02353265389067876051 ),
 .UNSPECIFIED. ) ;
#10966=CARTESIAN_POINT ( 'NONE',  ( 7.942924499382692183, 26.10933434278762988, 19.44382864746247819 ) ) ;
#10967=CARTESIAN_POINT ( 'NONE',  ( -2.509638519179916205, 54.33675374340515418, 20.85128429580866083 ) ) ;
#10968=CARTESIAN_POINT ( 'NONE',  ( 4.166436715168401861, 29.09658851243931821, -20.58482738948554314 ) ) ;
#10970=CARTESIAN_POINT ( 'NONE',  ( 2.571758291765529985E-15, 45.00000000000000711, 21.00000000000000000 ) ) ;
#10992=EDGE_CURVE ( 'NONE', #5152, #8715, #11514, .T. ) ;
#10996=CARTESIAN_POINT ( 'NONE',  ( -2.645619823791141467, 45.75416279094086036, 24.85999165416970413 ) ) ;
#11001=DIRECTION ( 'NONE',  ( -0.000000000000000000, -0.000000000000000000, 1.000000000000000000 ) ) ;
#11017=CARTESIAN_POINT ( 'NONE',  ( 4.452539714567801177, 11.03997247681473404, -24.60205477162727661 ) ) ;
#11059=CARTESIAN_POINT ( 'NONE',  ( -3.974987698915826595, 46.94954269600466290, 24.68264807992340337 ) ) ;
#11060=ORIENTED_EDGE ( 'NONE', *, *, #2173, .F. ) ;
#11077=CARTESIAN_POINT ( 'NONE',  ( -5.024407006007729493, 11.34777053809138003, -20.39219789878416478 ) ) ;
#11079=CARTESIAN_POINT ( 'NONE',  ( -6.608338170980154302, 27.53359326989389189, 24.11557641055247458 ) ) ;
#11083=CARTESIAN_POINT ( 'NONE',  ( -2.618974170005213153, 10.32668121623932400, 24.87084347637328108 ) ) ;
#11087=CARTESIAN_POINT ( 'NONE',  ( 8.664233696039474353, 25.03468766560890302, 23.45371044974007901 ) ) ;
#11088=CARTESIAN_POINT ( 'NONE',  ( 4.491162728695237583, 47.77810914732295799, 20.51453334527777628 ) ) ;
#11091=CARTESIAN_POINT ( 'NONE',  ( 2.216120825188211185, 45.50613141711284015, 24.90340997055814398 ) ) ;
#11100=ORIENTED_EDGE ( 'NONE', *, *, #640, .F. ) ;
#11138=ORIENTED_EDGE ( 'NONE', *, *, #10024, .F. ) ;
#11139=CARTESIAN_POINT ( 'NONE',  ( -5.017800233121429088, 11.34386344135788605, -24.49301625034288321 ) ) ;
#11140=CARTESIAN_POINT ( 'NONE',  ( 5.029111531688879921, 11.35041964440615914, -24.49069713376460555 ) ) ;
#11142=CARTESIAN_POINT ( 'NONE',  ( -6.609692946276023662, 12.48878433695339218, 24.11181729628509984 ) ) ;
#11145=CARTESIAN_POINT ( 'NONE',  ( -6.629750755640679394, 12.48603128090877057, 19.93185325444923706 ) ) ;
#11149=CARTESIAN_POINT ( 'NONE',  ( -3.973554925899839052, 53.05255087154787219, 24.68288788663009825 ) ) ;
#11162=CIRCLE ( 'NONE', #11373, 21.00000000000000000 ) ;
#11163=CARTESIAN_POINT ( 'NONE',  ( -3.594513446512490388E-16, 55.00000000000000000, -21.00000000000000000 ) ) ;
#11168=ADVANCED_FACE ( 'NONE', ( #5506 ), #9373, .F. ) ;
#11177=CARTESIAN_POINT ( 'NONE',  ( -5.029901707005755895, 28.64912781045596901, 20.39087425871785086 ) ) ;
#11184=FACE_OUTER_BOUND ( 'NONE', #8333, .T. ) ;
#11185=ORIENTED_EDGE ( 'NONE', *, *, #12344, .T. ) ;
#11199=CARTESIAN_POINT ( 'NONE',  ( -6.608660176926854923, 12.46713484822145190, -24.11541629257941111 ) ) ;
#11204=FACE_OUTER_BOUND ( 'NONE', #9162, .T. ) ;
#11257=B_SPLINE_CURVE_WITH_KNOTS ( 'NONE', 3,
 ( #6463, #7478, #10323, #11351, #6520, #5437, #2511, #1500, #9120, #3280, #9307, #6257, #6384, #2329, #6195, #11079, #3399, #2386, #12035, #4290, #5314, #9246, #3338, #11264, #10191, #7202, #428, #10135 ),
 .UNSPECIFIED., .F., .F.,
 ( 4, 2, 2, 2, 2, 2, 2, 2, 2, 2, 2, 2, 2, 4 ),
 ( 0.03159723681526421801, 0.03258403062298791120, 0.03357082443071160438, 0.03554441204615898381, 0.03653120585388267699, 0.03751799966160637018, 0.03850479346933006336, 0.03949158727705375654, 0.04146517489250114985, 0.04245196870022484303, 0.04343876250794853622, 0.04541235012339592259, 0.04639914393111962271, 0.04738593773884331589 ),
 .UNSPECIFIED. ) ;
#11264=CARTESIAN_POINT ( 'NONE',  ( -1.651830483015944262, 29.86811216670179903, 24.94746627493933744 ) ) ;
#11270=CARTESIAN_POINT ( 'NONE',  ( -8.963542696543054689, 15.55476857908299237, 18.99166849128095791 ) ) ;
#11274=DIRECTION ( 'NONE',  ( 0.000000000000000000, 1.000000000000000000, 0.000000000000000000 ) ) ;
#11281=VECTOR ( 'NONE', #1044, 1000.000000000000000 ) ;
#11286=DIRECTION ( 'NONE',  ( 0.000000000000000000, 0.000000000000000000, -1.000000000000000000 ) ) ;
#11293=VECTOR ( 'NONE', #11001, 1000.000000000000000 ) ;
#11300=B_SPLINE_CURVE_WITH_KNOTS ( 'NONE', 3,
 ( #7608, #1016, #5830, #3857, #5770, #4877, #9639, #8682, #6773, #7734, #10638, #9701, #8742, #4299, #11918, #8999, #10079, #12044, #10762, #9828, #10968, #376, #2073, #5004, #7985, #4176 ),
 .UNSPECIFIED., .F., .F.,
 ( 4, 2, 2, 2, 2, 2, 2, 2, 2, 2, 2, 2, 4 ),
 ( 0.04761567710518913032, 0.04860603727850610484, 0.04959639745182307935, 0.05157711779845704225, 0.05256747797177403064, 0.05355783814509101903, 0.05454819831840800742, 0.05553855849172499581, 0.05751927883835896566, 0.05850963901167595405, 0.05949999918499294244, 0.06148071953162691228, 0.06346143987826088906 ),
 .UNSPECIFIED. ) ;
#11306=VERTEX_POINT ( 'NONE', #9047 ) ;
#11322=CARTESIAN_POINT ( 'NONE',  ( 7.514434402675104430, 13.39403693888593772, 23.84492327520115396 ) ) ;
#11326=CARTESIAN_POINT ( 'NONE',  ( 1.615667985723896471, 54.74301895128219542, 20.93994550997156168 ) ) ;
#11335=CARTESIAN_POINT ( 'NONE',  ( 3.061616997868383043E-15, 139.9999999999999716, 25.00000000000000000 ) ) ;
#11336=CARTESIAN_POINT ( 'NONE',  ( 0.000000000000000000, 139.9999999999999716, -25.00000000000000000 ) ) ;
#11344=CARTESIAN_POINT ( 'NONE',  ( 0.6522419138580031195, 45.03179559853693092, 24.99358091562669060 ) ) ;
#11351=CARTESIAN_POINT ( 'NONE',  ( -9.918452521082530282, 21.31677563331469116, 22.94832388515032662 ) ) ;
#11373=AXIS2_PLACEMENT_3D ( 'NONE', #5848, #10781, #72 ) ;
#11387=CARTESIAN_POINT ( 'NONE',  ( 4.838482977639748661, 51.30270979396780717, 20.43510396060395706 ) ) ;
#11392=ORIENTED_EDGE ( 'NONE', *, *, #139, .T. ) ;
#11402=CARTESIAN_POINT ( 'NONE',  ( -9.934419958767060521, 21.32062905558055022, -18.50213348364253818 ) ) ;
#11410=CARTESIAN_POINT ( 'NONE',  ( -3.594513446512490388E-16, 55.00000000000000000, -21.00000000000000000 ) ) ;
#11416=EDGE_CURVE ( 'NONE', #2444, #11587, #4653, .T. ) ;
#11433=CARTESIAN_POINT ( 'NONE',  ( 0.000000000000000000, 0.000000000000000000, 0.000000000000000000 ) ) ;
#11443=ORIENTED_EDGE ( 'NONE', *, *, #8936, .F. ) ;
#11451=CARTESIAN_POINT ( 'NONE',  ( 5.854672968065819383, 11.88659906342193295, -20.16928711762458448 ) ) ;
#11455=CARTESIAN_POINT ( 'NONE',  ( -4.336320944401498956, 47.48960973344409098, 20.54824459866649988 ) ) ;
#11470=CARTESIAN_POINT ( 'NONE',  ( -4.735706364529653989, 51.61244378856764570, -20.45911749698736060 ) ) ;
#11483=DIRECTION ( 'NONE',  ( -0.000000000000000000, -0.000000000000000000, 1.000000000000000000 ) ) ;
#11485=ORIENTED_EDGE ( 'NONE', *, *, #9369, .F. ) ;
#11487=CARTESIAN_POINT ( 'NONE',  ( -0.3269246974466745170, 45.00000000000000000, -20.99999999999999289 ) ) ;
#11490=CARTESIAN_POINT ( 'NONE',  ( 10.00000000000000355, 20.00000000000000355, 18.46618531261938401 ) ) ;
#11502=CARTESIAN_POINT ( 'NONE',  ( -5.845037936402837531, 28.12045204670673826, -24.30869324251348829 ) ) ;
#11508=ORIENTED_EDGE ( 'NONE', *, *, #3401, .F. ) ;
#11510=CARTESIAN_POINT ( 'NONE',  ( 2.631235708468342871, 10.32974564483150814, -20.84467326578077362 ) ) ;
#11514=LINE ( 'NONE', #11335, #517 ) ;
#11531=EDGE_CURVE ( 'NONE', #6613, #1932, #2493, .T. ) ;
#11570=ORIENTED_EDGE ( 'NONE', *, *, #11969, .F. ) ;
#11574=B_SPLINE_CURVE_WITH_KNOTS ( 'NONE', 3,
 ( #3343, #8357, #10076, #10252, #7336, #10139, #7211, #8236, #12224, #3404, #3526, #8418, #11145, #1628, #4297, #1506, #7399, #11270, #4418, #2575, #1450, #6447, #9375, #12288, #2335, #6204 ),
 .UNSPECIFIED., .F., .F.,
 ( 4, 2, 2, 2, 2, 2, 2, 2, 2, 2, 2, 2, 4 ),
 ( 0.01588129651937168763, 0.01687311342740074882, 0.01786493033542981002, 0.01885674724345887468, 0.01984856415148793934, 0.02183219796754606173, 0.02381583178360418412, 0.02579946559966230998, 0.02679128250769137465, 0.02778309941572043584, 0.02877491632374950398, 0.02976673323177856517, 0.03175036704783668062 ),
 .UNSPECIFIED. ) ;
#11577=CARTESIAN_POINT ( 'NONE',  ( 9.102720968516898381, 15.84716940310434197, -18.92511261036585779 ) ) ;
#11587=VERTEX_POINT ( 'NONE', #11755 ) ;
#11589=CARTESIAN_POINT ( 'NONE',  ( 2.509213302053919570, 54.33723024690351622, -20.85136804008542555 ) ) ;
#11602=CARTESIAN_POINT ( 'NONE',  ( 0.6684871184501431918, 29.98311267939276092, -24.99323153604321490 ) ) ;
#11658=ORIENTED_EDGE ( 'NONE', *, *, #139, .F. ) ;
#11660=CARTESIAN_POINT ( 'NONE',  ( -6.117437525492237960, 27.91716672128773880, -20.09092915124056233 ) ) ;
#11671=CARTESIAN_POINT ( 'NONE',  ( 9.739799295956466096, 22.29052955100696920, -23.02479834983350671 ) ) ;
#11685=ORIENTED_EDGE ( 'NONE', *, *, #11811, .T. ) ;
#11686=DIRECTION ( 'NONE',  ( -0.000000000000000000, -0.000000000000000000, 1.000000000000000000 ) ) ;
#11697=CARTESIAN_POINT ( 'NONE',  ( 0.3267965066156393039, 44.99999999999999289, -25.00000000000000355 ) ) ;
#11698=VERTEX_POINT ( 'NONE', #3543 ) ;
#11705=ADVANCED_FACE ( 'NONE', ( #2658 ), #9391, .F. ) ;
#11714=FACE_OUTER_BOUND ( 'NONE', #10853, .T. ) ;
#11718=ORIENTED_EDGE ( 'NONE', *, *, #12103, .F. ) ;
#11726=CARTESIAN_POINT ( 'NONE',  ( 4.991728713179328203, 49.66892950866279932, -20.39811079091650114 ) ) ;
#11733=CARTESIAN_POINT ( 'NONE',  ( 7.942143053965557975, 26.11098614794844863, -23.70800582113895061 ) ) ;
#11743=ORIENTED_EDGE ( 'NONE', *, *, #9632, .T. ) ;
#11755=CARTESIAN_POINT ( 'NONE',  ( -10.00000000000000355, 20.00000000000000355, 22.91287847477919826 ) ) ;
#11761=ORIENTED_EDGE ( 'NONE', *, *, #12344, .F. ) ;
#11790=VERTEX_POINT ( 'NONE', #7228 ) ;
#11808=CARTESIAN_POINT ( 'NONE',  ( -2.507735966467860678, 54.33796433351858468, -24.87540749666489148 ) ) ;
#11811=EDGE_CURVE ( 'NONE', #2736, #11698, #3264, .T. ) ;
#11821=CARTESIAN_POINT ( 'NONE',  ( 3.764997658848628692, 46.69378447153945189, -24.71596740620162436 ) ) ;
#11833=CARTESIAN_POINT ( 'NONE',  ( -8.479561508268508518, 25.31046866060374967, 19.21289678253943478 ) ) ;
#11847=FACE_OUTER_BOUND ( 'NONE', #1839, .T. ) ;
#11856=CARTESIAN_POINT ( 'NONE',  ( 2.217259272193051967, 45.50669502826730195, 20.88480240601442262 ) ) ;
#11858=CARTESIAN_POINT ( 'NONE',  ( 2.571758278209441661E-15, 139.9999999999999716, 21.00000000000000000 ) ) ;
#11879=FACE_OUTER_BOUND ( 'NONE', #8758, .T. ) ;
#11894=EDGE_LOOP ( 'NONE', ( #2234, #2647 ) ) ;
#11905=CARTESIAN_POINT ( 'NONE',  ( 5.000000000000000000, 50.00000000000000000, -24.49489742783178414 ) ) ;
#11910=CARTESIAN_POINT ( 'NONE',  ( -5.305379791812843138, 11.51712698327468942, -20.32072021070228018 ) ) ;
#11916=CARTESIAN_POINT ( 'NONE',  ( -3.974640651900942512, 46.94910328357455143, -24.68270373814292640 ) ) ;
#11917=CARTESIAN_POINT ( 'NONE',  ( -4.999999999999999112, 50.32699065753391920, 20.39607805437114152 ) ) ;
#11918=CARTESIAN_POINT ( 'NONE',  ( 7.302632803679189877, 26.83934157082542882, -19.69087995796197887 ) ) ;
#11930=CARTESIAN_POINT ( 'NONE',  ( 0.000000000000000000, 139.9999999999999716, 0.000000000000000000 ) ) ;
#11969=EDGE_CURVE ( 'NONE', #4011, #5701, #10506, .T. ) ;
#11970=VERTEX_POINT ( 'NONE', #5951 ) ;
#11972=CARTESIAN_POINT ( 'NONE',  ( 9.868114579493717287, 18.34823788458374594, -22.97009550651098309 ) ) ;
#11980=CARTESIAN_POINT ( 'NONE',  ( -5.000000000000000888, 49.67303160952345564, -24.49489742783178059 ) ) ;
#11987=CARTESIAN_POINT ( 'NONE',  ( 3.061565168526138680E-15, 55.00000000000000000, 25.00000000000000000 ) ) ;
#12012=ORIENTED_EDGE ( 'NONE', *, *, #4287, .T. ) ;
#12017=EDGE_CURVE ( 'NONE', #7940, #2752, #5978, .T. ) ;
#12032=CARTESIAN_POINT ( 'NONE',  ( -9.349016511544222752, 16.43577148148449396, -18.80467678224717432 ) ) ;
#12035=CARTESIAN_POINT ( 'NONE',  ( -5.025242304149237782, 28.65182443915274746, 24.49149081028624053 ) ) ;
#12044=CARTESIAN_POINT ( 'NONE',  ( 5.316967106970424517, 28.47548153940854831, -20.31764798226379654 ) ) ;
#12050=LINE ( 'NONE', #11858, #12324 ) ;
#12089=ORIENTED_EDGE ( 'NONE', *, *, #3433, .F. ) ;
#12103=EDGE_CURVE ( 'NONE', #7957, #2444, #11574, .T. ) ;
#12107=CARTESIAN_POINT ( 'NONE',  ( 3.547335893868845513, 29.35536450536750408, 24.74892486337281738 ) ) ;
#12108=CARTESIAN_POINT ( 'NONE',  ( -3.306342958134543153, 53.76488593550792672, 24.78149064010515445 ) ) ;
#12109=ORIENTED_EDGE ( 'NONE', *, *, #985, .F. ) ;
#12132=CARTESIAN_POINT ( 'NONE',  ( -7.926973682980901437, 26.10475523195332315, 19.44767585397084986 ) ) ;
#12136=CARTESIAN_POINT ( 'NONE',  ( -2.505953076466797658, 45.67021871533034982, 24.87450930309000441 ) ) ;
#12158=CARTESIAN_POINT ( 'NONE',  ( -7.295229519525479489, 13.15279342069419499, -23.91310413417861369 ) ) ;
#12169=DIRECTION ( 'NONE',  ( 0.000000000000000000, 0.000000000000000000, 1.000000000000000000 ) ) ;
#12174=CARTESIAN_POINT ( 'NONE',  ( 3.764018802651051487, 53.30721710162806204, 24.71610890024348350 ) ) ;
#12183=ORIENTED_EDGE ( 'NONE', *, *, #9402, .T. ) ;
#12220=CARTESIAN_POINT ( 'NONE',  ( 0.000000000000000000, 139.9999999999999716, -25.00000000000000000 ) ) ;
#12224=CARTESIAN_POINT ( 'NONE',  ( -3.567631371761228909, 10.65224600664762455, 20.69704057926737661 ) ) ;
#12228=AXIS2_PLACEMENT_3D ( 'NONE', #8358, #6448, #6205 ) ;
#12232=CARTESIAN_POINT ( 'NONE',  ( 5.000000000000000000, 49.66865400565588828, 24.49489742783178414 ) ) ;
#12254=CARTESIAN_POINT ( 'NONE',  ( -7.296251494991419229, 26.84606392143152220, 19.69323068918331288 ) ) ;
#12259=CARTESIAN_POINT ( 'NONE',  ( -2.510602112304970213, 45.66379892316987821, -20.85116850286192403 ) ) ;
#12262=CARTESIAN_POINT ( 'NONE',  ( 3.252657063245354863, 10.53797398869742352, 20.74903557764927697 ) ) ;
#12284=CARTESIAN_POINT ( 'NONE',  ( 0.3297592447147374983, 55.00000000000001421, 21.00000000000000711 ) ) ;
#12286=CARTESIAN_POINT ( 'NONE',  ( 0.000000000000000000, 20.00000000000000355, -28.00000000000000711 ) ) ;
#12288=CARTESIAN_POINT ( 'NONE',  ( -9.935036394566825635, 18.68123011217310392, 18.50181441894565637 ) ) ;
#12291=CARTESIAN_POINT ( 'NONE',  ( 7.931687869515056555, 26.09867752937626406, 23.70939416258605803 ) ) ;
#12292=CARTESIAN_POINT ( 'NONE',  ( 3.061565168526138680E-15, 55.00000000000000000, 25.00000000000000000 ) ) ;
#12324=VECTOR ( 'NONE', #7154, 1000.000000000000000 ) ;
#12342=CARTESIAN_POINT ( 'NONE',  ( 4.490845867985273188, 52.22224976665338403, 20.51459889515917467 ) ) ;
#12344=EDGE_CURVE ( 'NONE', #7546, #3410, #8271, .T. ) ;
#12354=CARTESIAN_POINT ( 'NONE',  ( -0.3301821175306443035, 55.00000000000001421, 25.00000000000000000 ) ) ;
#12370=AXIS2_PLACEMENT_3D ( 'NONE', #2455, #11274, #12169 ) ;
#12384=CARTESIAN_POINT ( 'NONE',  ( -2.217721585883460023, 45.50683808975505684, -20.88476930822203315 ) ) ;
#12396=ORIENTED_EDGE ( 'NONE', *, *, #2398, .T. ) ;
#12407=DIRECTION ( 'NONE',  ( -0.000000000000000000, -1.000000000000000000, -0.000000000000000000 ) ) ;
#12408=CARTESIAN_POINT ( 'NONE',  ( -3.051733061893640908, 46.02601656636597482, 20.77886321925161894 ) ) ;
#12417=VECTOR ( 'NONE', #9214, 1000.000000000000000 ) ;
#12424=AXIS2_PLACEMENT_3D ( 'NONE', #6390, #7212, #555 ) ;
#12444=CARTESIAN_POINT ( 'NONE',  ( -10.00000000000000355, 20.00000000000000355, 18.46618531261938756 ) ) ;
#12446=CARTESIAN_POINT ( 'NONE',  ( 9.349263383750175294, 16.43657559142555868, 18.80454793984171147 ) ) ;
#12449=DIRECTION ( 'NONE',  ( 0.000000000000000000, 1.000000000000000000, 0.000000000000000000 ) ) ;
#12450=CARTESIAN_POINT ( 'NONE',  ( 3.061616998149962604E-15, 10.00000000000000000, 25.00000000000000000 ) ) ;
#12476=CARTESIAN_POINT ( 'NONE',  ( 1.620915035299892226, 54.74117664902413338, -20.93952827735066791 ) ) ;
#12479=CARTESIAN_POINT ( 'NONE',  ( -6.616163141694259231, 27.50539512973521283, -19.93225680451049087 ) ) ;
#12484=CARTESIAN_POINT ( 'NONE',  ( -4.968127171134807618, 50.65287670289590949, -20.40397231773725650 ) ) ;
#12506=CARTESIAN_POINT ( 'NONE',  ( 8.663040577955531063, 14.96273206212219975, 19.13393308409949967 ) ) ;
#12518=CARTESIAN_POINT ( 'NONE',  ( -10.00000000000000355, 20.00000000000000355, -22.91287847477919826 ) ) ;
#12526=CARTESIAN_POINT ( 'NONE',  ( 8.653685250178629218, 14.97800528606349424, -19.13485699315961597 ) ) ;
#12540=VERTEX_POINT ( 'NONE', #7439 ) ;
#12578=COLOUR_RGB('Grey',0.48,0.52,0.57);
#12579=FILL_AREA_STYLE_COLOUR('',#12578);
#12580=FILL_AREA_STYLE('',(#12579));
#12581=SURFACE_STYLE_FILL_AREA(#12580);
#12582=SURFACE_SIDE_STYLE('',(#12581));
#12583=SURFACE_STYLE_USAGE(.BOTH.,#12582);
#12584=PRESENTATION_STYLE_ASSIGNMENT((#12583));
ENDSEC;
END-ISO-10303-21;
